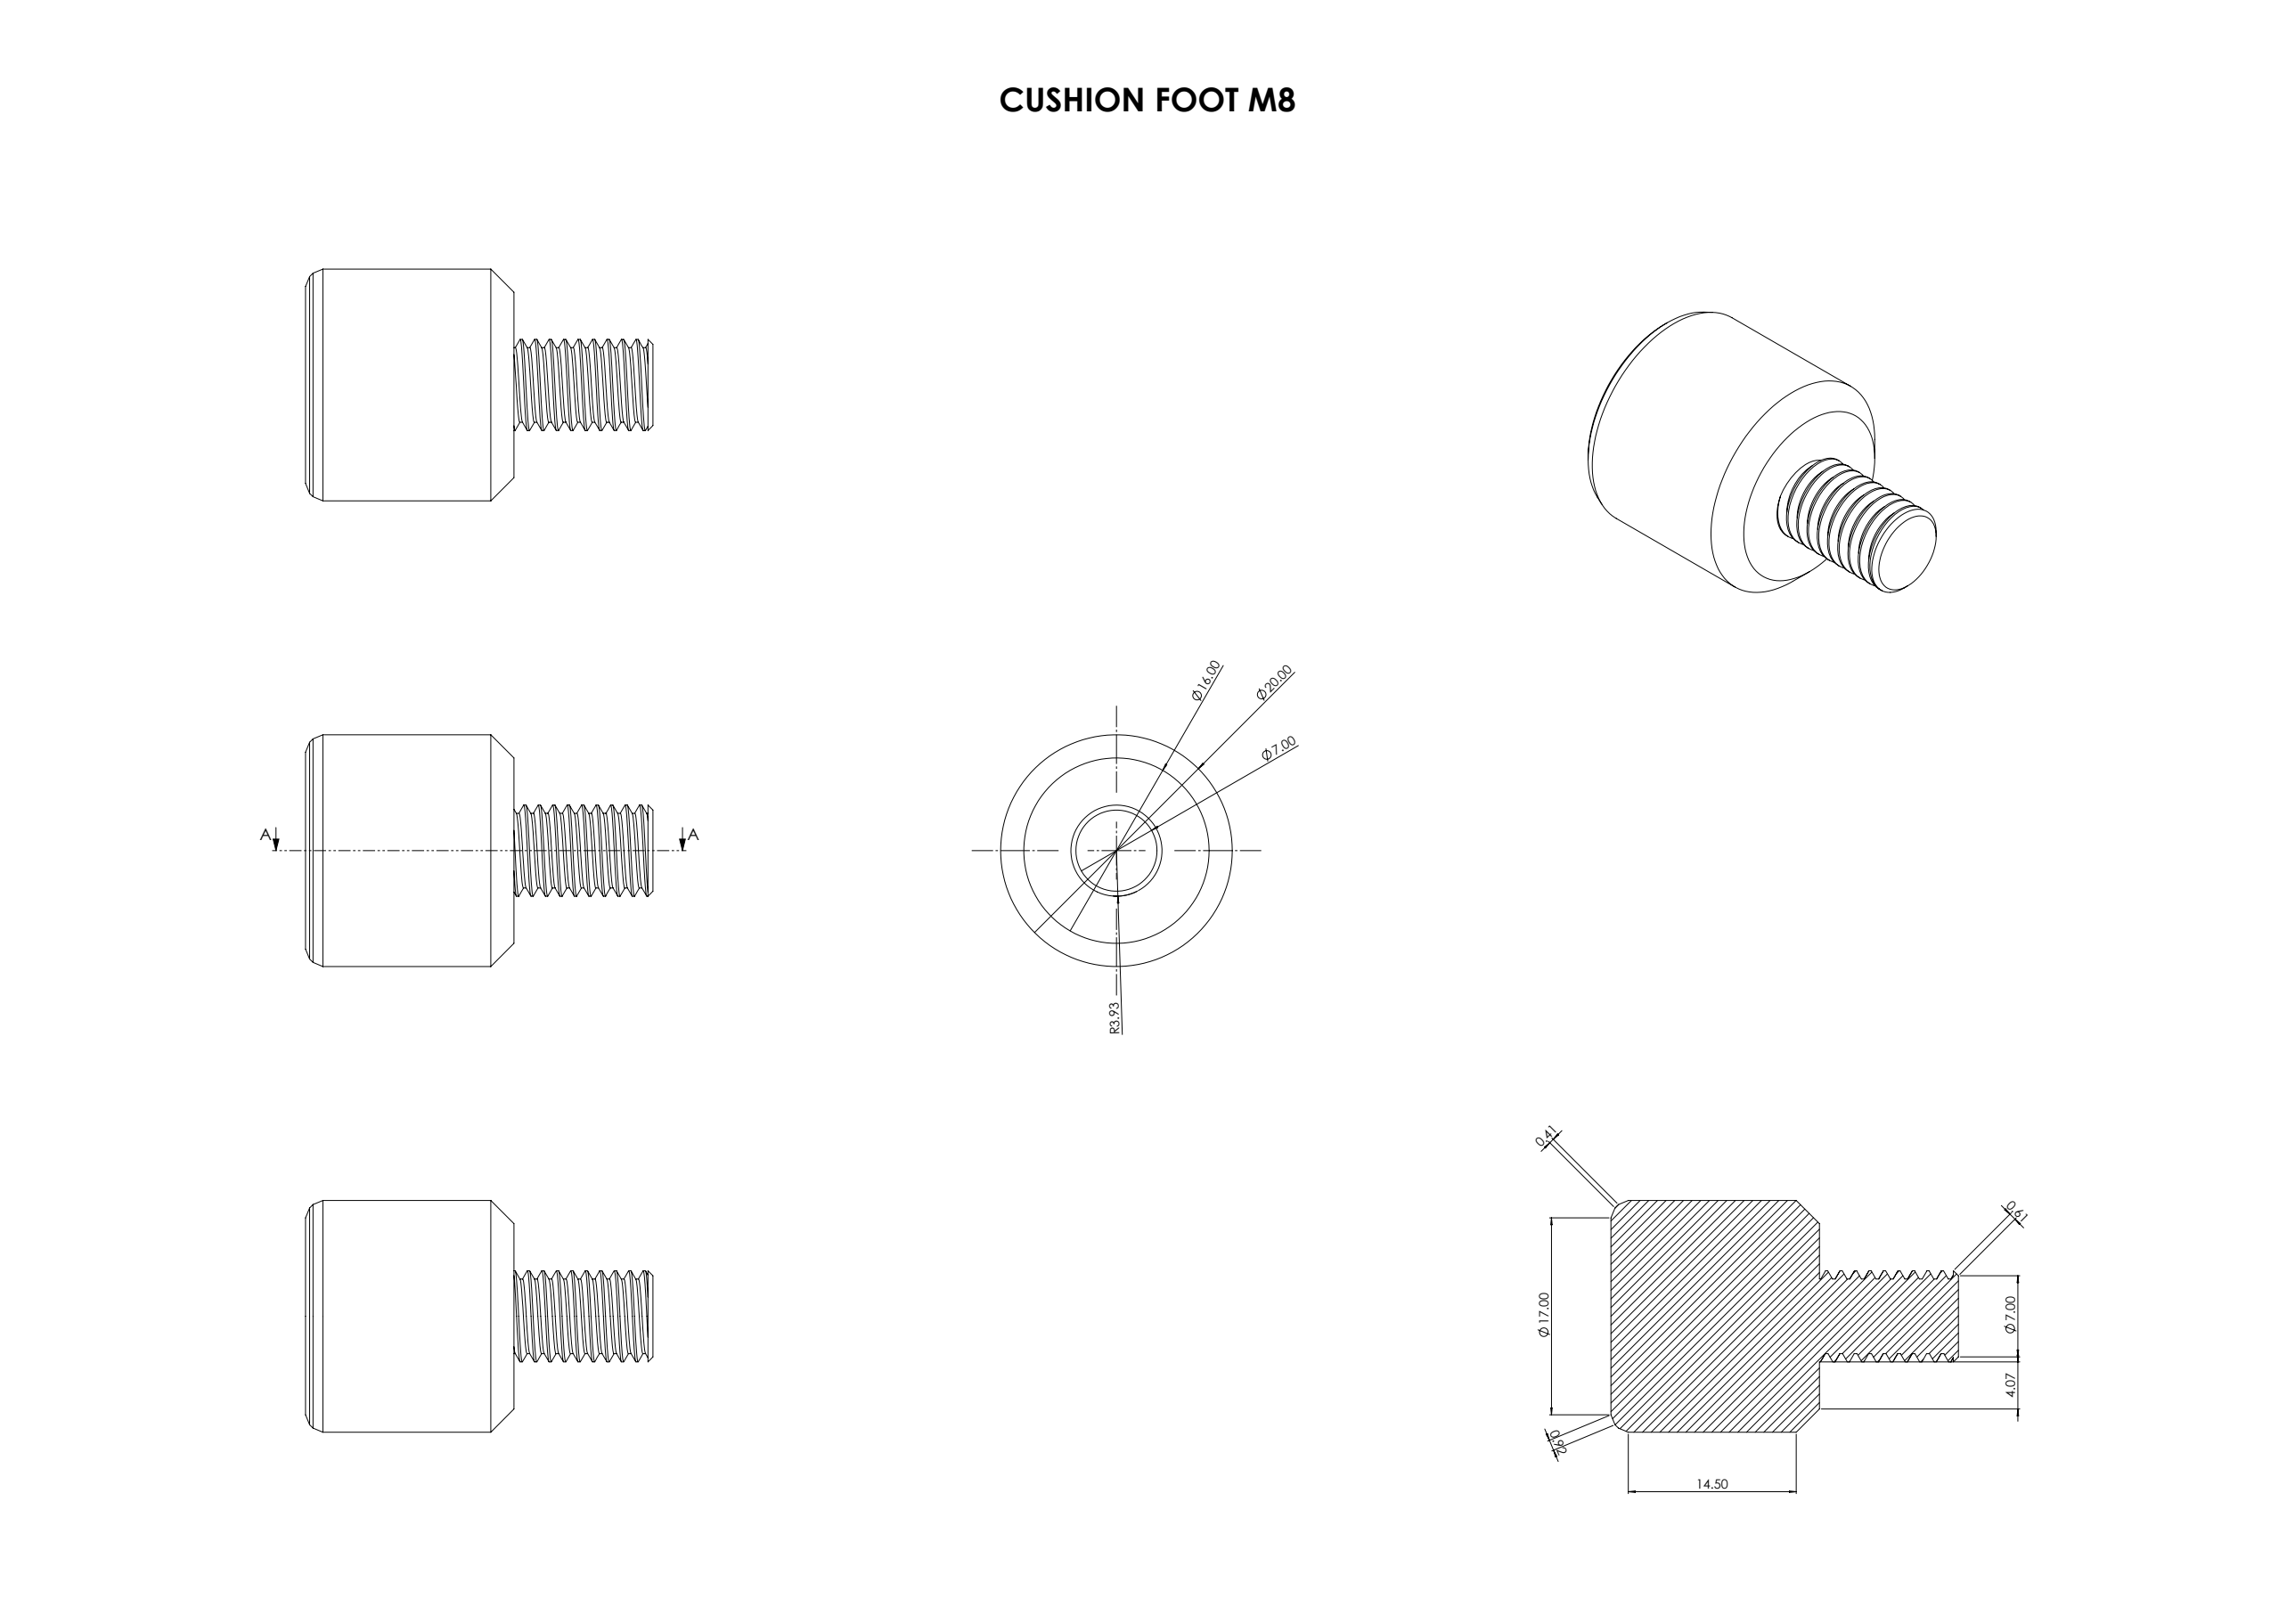
ISO-10303-21;
HEADER;
/* Generated by software containing ST-Developer
 * from STEP Tools, Inc. (www.steptools.com) 
 */

FILE_DESCRIPTION(
/* description */ (''),
/* implementation_level */ '2;1');

FILE_NAME(
/* name */ '15_Cushion_Foot_M8.step',
/* time_stamp */ '2026-10-26T06:13:19-07:00',
/* author */ (''),
/* organization */ (''),
/* preprocessor_version */ 'ST-DEVELOPER v20.2',
/* originating_system */ 'Autodesk Translation Framework v15.15.0.0',
/* authorisation */ '');

FILE_SCHEMA (('AUTOMOTIVE_DESIGN { 1 0 10303 214 3 1 1 }','TECHNICAL_DATA_PACKAGING'));
ENDSEC;

DATA;
#10=MECHANICAL_DESIGN_GEOMETRIC_PRESENTATION_REPRESENTATION('',(#313),#56639);
#273=SHAPE_REPRESENTATION_RELATIONSHIP('SRR','None',#56761,#293);
#293=ADVANCED_BREP_SHAPE_REPRESENTATION('',(#333),#56635);
#313=STYLED_ITEM('',(#56929),#333);
#333=MANIFOLD_SOLID_BREP('Body1',#16965);
#355=B_SPLINE_SURFACE_WITH_KNOTS('',3,3,((#37649,#37650,#37651,#37652,#37653,
#37654,#37655,#37656,#37657,#37658,#37659,#37660,#37661,#37662,#37663,#37664,
#37665,#37666,#37667,#37668,#37669,#37670,#37671,#37672,#37673,#37674,#37675,
#37676,#37677,#37678,#37679,#37680,#37681,#37682,#37683,#37684,#37685,#37686,
#37687,#37688,#37689,#37690,#37691,#37692,#37693,#37694,#37695,#37696,#37697,
#37698,#37699,#37700,#37701,#37702,#37703,#37704,#37705,#37706,#37707,#37708,
#37709,#37710,#37711,#37712),(#37713,#37714,#37715,#37716,#37717,#37718,
#37719,#37720,#37721,#37722,#37723,#37724,#37725,#37726,#37727,#37728,#37729,
#37730,#37731,#37732,#37733,#37734,#37735,#37736,#37737,#37738,#37739,#37740,
#37741,#37742,#37743,#37744,#37745,#37746,#37747,#37748,#37749,#37750,#37751,
#37752,#37753,#37754,#37755,#37756,#37757,#37758,#37759,#37760,#37761,#37762,
#37763,#37764,#37765,#37766,#37767,#37768,#37769,#37770,#37771,#37772,#37773,
#37774,#37775,#37776),(#37777,#37778,#37779,#37780,#37781,#37782,#37783,
#37784,#37785,#37786,#37787,#37788,#37789,#37790,#37791,#37792,#37793,#37794,
#37795,#37796,#37797,#37798,#37799,#37800,#37801,#37802,#37803,#37804,#37805,
#37806,#37807,#37808,#37809,#37810,#37811,#37812,#37813,#37814,#37815,#37816,
#37817,#37818,#37819,#37820,#37821,#37822,#37823,#37824,#37825,#37826,#37827,
#37828,#37829,#37830,#37831,#37832,#37833,#37834,#37835,#37836,#37837,#37838,
#37839,#37840),(#37841,#37842,#37843,#37844,#37845,#37846,#37847,#37848,
#37849,#37850,#37851,#37852,#37853,#37854,#37855,#37856,#37857,#37858,#37859,
#37860,#37861,#37862,#37863,#37864,#37865,#37866,#37867,#37868,#37869,#37870,
#37871,#37872,#37873,#37874,#37875,#37876,#37877,#37878,#37879,#37880,#37881,
#37882,#37883,#37884,#37885,#37886,#37887,#37888,#37889,#37890,#37891,#37892,
#37893,#37894,#37895,#37896,#37897,#37898,#37899,#37900,#37901,#37902,#37903,
#37904)),.UNSPECIFIED.,.F.,.F.,.F.,(4,4),(4,1,1,1,1,1,1,1,1,1,1,1,1,1,1,
1,1,1,1,1,1,1,1,1,1,1,1,1,1,1,1,1,1,1,1,1,1,1,1,1,1,1,1,1,1,1,1,1,1,1,1,
1,1,1,1,1,1,1,1,1,1,4),(0.,0.0820126057383863),(8.31473274985799,9.30167185077656,
10.2886109516951,11.2755500526137,12.2624891535323,13.2494282544508,14.2363673553694,
15.223306456288,16.2102455572066,17.1971846581251,18.1841237590437,19.1710628599623,
20.1580019608808,21.1449410617994,22.131880162718,23.1188192636365,24.1057583645551,
25.0926974654737,26.0796365663922,27.0665756673108,28.0535147682294,29.040453869148,
30.0273929700665,31.0143320709851,32.0012711719037,32.9882102728222,33.9751493737408,
34.9620884746594,35.9490275755779,36.9359666764965,37.9229057774151,38.9098448783337,
39.8967839792522,40.8837230801708,41.8706621810894,42.8576012820079,43.8445403829265,
44.8314794838451,45.8184185847636,46.8053576856822,47.7922967866008,48.7792358875193,
49.7661749884379,50.7531140893565,51.7400531902751,52.7269922911936,53.7139313921122,
54.7008704930308,55.6878095939493,56.6747486948679,57.6616877957865,58.6486268967051,
59.6355659976236,60.6225050985422,61.6094441994608,62.5963833003793,63.5833224012979,
64.5702615022165,65.557200603135,66.5441397040536,67.5310788049722,68.5180179058908),
 .UNSPECIFIED.);
#356=B_SPLINE_SURFACE_WITH_KNOTS('',3,3,((#38027,#38028,#38029,#38030,#38031,
#38032,#38033,#38034,#38035,#38036,#38037,#38038,#38039,#38040,#38041,#38042,
#38043,#38044,#38045,#38046,#38047,#38048,#38049,#38050,#38051,#38052,#38053,
#38054,#38055,#38056,#38057,#38058,#38059,#38060,#38061,#38062,#38063,#38064,
#38065,#38066,#38067,#38068,#38069,#38070,#38071,#38072,#38073,#38074,#38075,
#38076,#38077,#38078,#38079,#38080,#38081,#38082,#38083,#38084,#38085,#38086,
#38087,#38088,#38089,#38090),(#38091,#38092,#38093,#38094,#38095,#38096,
#38097,#38098,#38099,#38100,#38101,#38102,#38103,#38104,#38105,#38106,#38107,
#38108,#38109,#38110,#38111,#38112,#38113,#38114,#38115,#38116,#38117,#38118,
#38119,#38120,#38121,#38122,#38123,#38124,#38125,#38126,#38127,#38128,#38129,
#38130,#38131,#38132,#38133,#38134,#38135,#38136,#38137,#38138,#38139,#38140,
#38141,#38142,#38143,#38144,#38145,#38146,#38147,#38148,#38149,#38150,#38151,
#38152,#38153,#38154),(#38155,#38156,#38157,#38158,#38159,#38160,#38161,
#38162,#38163,#38164,#38165,#38166,#38167,#38168,#38169,#38170,#38171,#38172,
#38173,#38174,#38175,#38176,#38177,#38178,#38179,#38180,#38181,#38182,#38183,
#38184,#38185,#38186,#38187,#38188,#38189,#38190,#38191,#38192,#38193,#38194,
#38195,#38196,#38197,#38198,#38199,#38200,#38201,#38202,#38203,#38204,#38205,
#38206,#38207,#38208,#38209,#38210,#38211,#38212,#38213,#38214,#38215,#38216,
#38217,#38218),(#38219,#38220,#38221,#38222,#38223,#38224,#38225,#38226,
#38227,#38228,#38229,#38230,#38231,#38232,#38233,#38234,#38235,#38236,#38237,
#38238,#38239,#38240,#38241,#38242,#38243,#38244,#38245,#38246,#38247,#38248,
#38249,#38250,#38251,#38252,#38253,#38254,#38255,#38256,#38257,#38258,#38259,
#38260,#38261,#38262,#38263,#38264,#38265,#38266,#38267,#38268,#38269,#38270,
#38271,#38272,#38273,#38274,#38275,#38276,#38277,#38278,#38279,#38280,#38281,
#38282)),.UNSPECIFIED.,.F.,.F.,.F.,(4,4),(4,1,1,1,1,1,1,1,1,1,1,1,1,1,1,
1,1,1,1,1,1,1,1,1,1,1,1,1,1,1,1,1,1,1,1,1,1,1,1,1,1,1,1,1,1,1,1,1,1,1,1,
1,1,1,1,1,1,1,1,1,1,4),(0.,0.0820126057383863),(11.6152142277547,12.6021533286733,
13.5890924295918,14.5760315305104,15.562970631429,16.5499097323475,17.5368488332661,
18.5237879341847,19.5107270351033,20.4976661360218,21.4846052369404,22.471544337859,
23.4584834387775,24.4454225396961,25.4323616406147,26.4193007415332,27.4062398424518,
28.3931789433704,29.380118044289,30.3670571452075,31.3539962461261,32.3409353470447,
33.3278744479632,34.3148135488818,35.3017526498004,36.2886917507189,37.2756308516375,
38.2625699525561,39.2495090534747,40.2364481543932,41.2233872553118,42.2103263562304,
43.1972654571489,44.1842045580675,45.1711436589861,46.1580827599046,47.1450218608232,
48.1319609617418,49.1189000626604,50.1058391635789,51.0927782644975,52.0797173654161,
53.0666564663346,54.0535955672532,55.0405346681718,56.0274737690903,57.0144128700089,
58.0013519709275,58.9882910718461,59.9752301727646,60.9621692736832,61.9491083746018,
62.9360474755203,63.9229865764389,64.9099256773575,65.8968647782761,66.8838038791946,
67.8707429801132,68.8576820810318,69.8446211819503,70.8315602828689,71.8184993837875),
 .UNSPECIFIED.);
#559=FACE_BOUND('',#3561,.T.);
#643=CONICAL_SURFACE('',#18350,9.82322330470336,0.392699081698723);
#644=CONICAL_SURFACE('',#18355,9.5,0.785398163397448);
#645=CONICAL_SURFACE('',#18360,8.92677669529664,1.17809724509617);
#646=CONICAL_SURFACE('',#18369,9.,0.785398163397448);
#647=CONICAL_SURFACE('',#18372,3.75,0.785398163397451);
#1180=CIRCLE('',#18329,3.933);
#1181=CIRCLE('',#18339,3.933);
#1182=CIRCLE('',#18341,3.22275);
#1183=CIRCLE('',#18351,10.);
#1184=CIRCLE('',#18352,10.);
#1185=CIRCLE('',#18353,9.64644660940673);
#1186=CIRCLE('',#18354,9.64644660940673);
#1187=CIRCLE('',#18356,9.35355339059327);
#1188=CIRCLE('',#18357,9.35355339059327);
#1189=CIRCLE('',#18359,10.);
#1190=CIRCLE('',#18361,8.5);
#1191=CIRCLE('',#18364,3.933);
#1192=CIRCLE('',#18366,3.22275);
#1193=CIRCLE('',#18368,3.933);
#1194=CIRCLE('',#18370,8.);
#1195=CIRCLE('',#18373,3.5);
#1470=CYLINDRICAL_SURFACE('',#18328,3.933);
#1471=CYLINDRICAL_SURFACE('',#18330,3.933);
#1472=CYLINDRICAL_SURFACE('',#18331,3.933);
#1473=CYLINDRICAL_SURFACE('',#18332,3.933);
#1474=CYLINDRICAL_SURFACE('',#18333,3.933);
#1475=CYLINDRICAL_SURFACE('',#18334,3.933);
#1476=CYLINDRICAL_SURFACE('',#18335,3.933);
#1477=CYLINDRICAL_SURFACE('',#18336,3.933);
#1478=CYLINDRICAL_SURFACE('',#18337,3.933);
#1479=CYLINDRICAL_SURFACE('',#18338,3.933);
#1480=CYLINDRICAL_SURFACE('',#18340,3.22275);
#1481=CYLINDRICAL_SURFACE('',#18342,3.22275);
#1482=CYLINDRICAL_SURFACE('',#18343,3.22275);
#1483=CYLINDRICAL_SURFACE('',#18344,3.22275);
#1484=CYLINDRICAL_SURFACE('',#18345,3.22275);
#1485=CYLINDRICAL_SURFACE('',#18346,3.22275);
#1486=CYLINDRICAL_SURFACE('',#18347,3.22275);
#1487=CYLINDRICAL_SURFACE('',#18348,3.22275);
#1488=CYLINDRICAL_SURFACE('',#18349,3.22275);
#1489=CYLINDRICAL_SURFACE('',#18358,10.);
#1490=CYLINDRICAL_SURFACE('',#18365,3.22275);
#1491=CYLINDRICAL_SURFACE('',#18367,3.933);
#2412=FACE_OUTER_BOUND('',#3530,.T.);
#2413=FACE_OUTER_BOUND('',#3531,.T.);
#2414=FACE_OUTER_BOUND('',#3532,.T.);
#2415=FACE_OUTER_BOUND('',#3533,.T.);
#2416=FACE_OUTER_BOUND('',#3534,.T.);
#2417=FACE_OUTER_BOUND('',#3535,.T.);
#2418=FACE_OUTER_BOUND('',#3536,.T.);
#2419=FACE_OUTER_BOUND('',#3537,.T.);
#2420=FACE_OUTER_BOUND('',#3538,.T.);
#2421=FACE_OUTER_BOUND('',#3539,.T.);
#2422=FACE_OUTER_BOUND('',#3540,.T.);
#2423=FACE_OUTER_BOUND('',#3541,.T.);
#2424=FACE_OUTER_BOUND('',#3542,.T.);
#2425=FACE_OUTER_BOUND('',#3543,.T.);
#2426=FACE_OUTER_BOUND('',#3544,.T.);
#2427=FACE_OUTER_BOUND('',#3545,.T.);
#2428=FACE_OUTER_BOUND('',#3546,.T.);
#2429=FACE_OUTER_BOUND('',#3547,.T.);
#2430=FACE_OUTER_BOUND('',#3548,.T.);
#2431=FACE_OUTER_BOUND('',#3549,.T.);
#2432=FACE_OUTER_BOUND('',#3550,.T.);
#2433=FACE_OUTER_BOUND('',#3551,.T.);
#2434=FACE_OUTER_BOUND('',#3552,.T.);
#2435=FACE_OUTER_BOUND('',#3553,.T.);
#2436=FACE_OUTER_BOUND('',#3554,.T.);
#2437=FACE_OUTER_BOUND('',#3555,.T.);
#2438=FACE_OUTER_BOUND('',#3556,.T.);
#2439=FACE_OUTER_BOUND('',#3557,.T.);
#2440=FACE_OUTER_BOUND('',#3558,.T.);
#2441=FACE_OUTER_BOUND('',#3559,.T.);
#2442=FACE_OUTER_BOUND('',#3560,.T.);
#2443=FACE_OUTER_BOUND('',#3562,.T.);
#2444=FACE_OUTER_BOUND('',#3563,.T.);
#3530=EDGE_LOOP('',(#13640,#13641,#13642,#13643));
#3531=EDGE_LOOP('',(#13644,#13645,#13646,#13647));
#3532=EDGE_LOOP('',(#13648,#13649,#13650,#13651));
#3533=EDGE_LOOP('',(#13652,#13653,#13654,#13655));
#3534=EDGE_LOOP('',(#13656,#13657,#13658,#13659));
#3535=EDGE_LOOP('',(#13660,#13661,#13662,#13663));
#3536=EDGE_LOOP('',(#13664,#13665,#13666,#13667));
#3537=EDGE_LOOP('',(#13668,#13669,#13670,#13671));
#3538=EDGE_LOOP('',(#13672,#13673,#13674,#13675));
#3539=EDGE_LOOP('',(#13676,#13677,#13678,#13679,#13680));
#3540=EDGE_LOOP('',(#13681,#13682,#13683,#13684));
#3541=EDGE_LOOP('',(#13685,#13686,#13687,#13688));
#3542=EDGE_LOOP('',(#13689,#13690,#13691,#13692));
#3543=EDGE_LOOP('',(#13693,#13694,#13695,#13696));
#3544=EDGE_LOOP('',(#13697,#13698,#13699,#13700));
#3545=EDGE_LOOP('',(#13701,#13702,#13703,#13704));
#3546=EDGE_LOOP('',(#13705,#13706,#13707,#13708));
#3547=EDGE_LOOP('',(#13709,#13710,#13711,#13712));
#3548=EDGE_LOOP('',(#13713,#13714,#13715,#13716));
#3549=EDGE_LOOP('',(#13717,#13718,#13719,#13720,#13721,#13722));
#3550=EDGE_LOOP('',(#13723,#13724,#13725,#13726,#13727,#13728));
#3551=EDGE_LOOP('',(#13729,#13730,#13731,#13732,#13733));
#3552=EDGE_LOOP('',(#13734,#13735,#13736,#13737,#13738));
#3553=EDGE_LOOP('',(#13739));
#3554=EDGE_LOOP('',(#13740,#13741,#13742,#13743));
#3555=EDGE_LOOP('',(#13744,#13745,#13746,#13747,#13748,#13749,#13750,#13751,
#13752,#13753,#13754,#13755,#13756,#13757,#13758,#13759,#13760,#13761,#13762,
#13763,#13764,#13765,#13766));
#3556=EDGE_LOOP('',(#13767,#13768,#13769,#13770));
#3557=EDGE_LOOP('',(#13771,#13772,#13773,#13774,#13775,#13776,#13777,#13778,
#13779,#13780,#13781,#13782,#13783,#13784,#13785,#13786,#13787,#13788,#13789,
#13790,#13791,#13792));
#3558=EDGE_LOOP('',(#13793,#13794,#13795));
#3559=EDGE_LOOP('',(#13796,#13797,#13798,#13799));
#3560=EDGE_LOOP('',(#13800));
#3561=EDGE_LOOP('',(#13801,#13802,#13803,#13804));
#3562=EDGE_LOOP('',(#13805,#13806,#13807,#13808,#13809,#13810));
#3563=EDGE_LOOP('',(#13811));
#4515=LINE('',#36739,#5469);
#4516=LINE('',#36763,#5470);
#4517=LINE('',#36811,#5471);
#4518=LINE('',#36859,#5472);
#4519=LINE('',#36913,#5473);
#4520=LINE('',#36961,#5474);
#4521=LINE('',#37009,#5475);
#4522=LINE('',#37063,#5476);
#4523=LINE('',#37111,#5477);
#4524=LINE('',#37165,#5478);
#4525=LINE('',#37212,#5479);
#4526=LINE('',#37232,#5480);
#4527=LINE('',#37257,#5481);
#4528=LINE('',#37282,#5482);
#4529=LINE('',#37307,#5483);
#4530=LINE('',#37332,#5484);
#4531=LINE('',#37356,#5485);
#4532=LINE('',#37381,#5486);
#4533=LINE('',#37406,#5487);
#4534=LINE('',#37433,#5488);
#4535=LINE('',#37439,#5489);
#4536=LINE('',#37446,#5490);
#4537=LINE('',#37449,#5491);
#4538=LINE('',#38385,#5492);
#4539=LINE('',#38390,#5493);
#5469=VECTOR('',#21681,4.);
#5470=VECTOR('',#21686,4.);
#5471=VECTOR('',#21689,4.);
#5472=VECTOR('',#21692,4.);
#5473=VECTOR('',#21695,4.);
#5474=VECTOR('',#21698,4.);
#5475=VECTOR('',#21701,4.);
#5476=VECTOR('',#21704,4.);
#5477=VECTOR('',#21707,4.);
#5478=VECTOR('',#21710,4.);
#5479=VECTOR('',#21715,3.22275);
#5480=VECTOR('',#21720,3.22275);
#5481=VECTOR('',#21723,3.22275);
#5482=VECTOR('',#21726,3.22275);
#5483=VECTOR('',#21729,3.22275);
#5484=VECTOR('',#21732,3.22275);
#5485=VECTOR('',#21735,3.22275);
#5486=VECTOR('',#21738,3.22275);
#5487=VECTOR('',#21741,3.22275);
#5488=VECTOR('',#21748,9.82322330470336);
#5489=VECTOR('',#21755,9.5);
#5490=VECTOR('',#21764,10.);
#5491=VECTOR('',#21767,8.92677669529664);
#5492=VECTOR('',#21788,9.);
#5493=VECTOR('',#21795,3.75);
#6085=B_SPLINE_CURVE_WITH_KNOTS('',3,(#36741,#36742,#36743,#36744,#36745,
#36746,#36747,#36748,#36749,#36750),.UNSPECIFIED.,.F.,.F.,(4,3,3,4),(-4.09274904019423,
-3.94775640367428,-2.96081730275571,-2.06120159751578),.UNSPECIFIED.);
#6086=B_SPLINE_CURVE_WITH_KNOTS('',3,(#36753,#36754,#36755,#36756,#36757,
#36758,#36759),.UNSPECIFIED.,.F.,.F.,(4,3,4),(0.,0.986939100918566,1.11004521091131),
 .UNSPECIFIED.);
#6087=B_SPLINE_CURVE_WITH_KNOTS('',3,(#36764,#36765,#36766,#36767,#36768,
#36769,#36770,#36771,#36772,#36773,#36774,#36775,#36776,#36777,#36778,#36779,
#36780,#36781,#36782,#36783,#36784,#36785),.UNSPECIFIED.,.F.,.F.,(4,3,3,
3,3,3,3,4),(-10.3759343473738,-9.8693910091857,-8.88245190826713,-7.89551280734856,
-6.90857370642999,-5.92163460551142,-4.93469550459285,-4.09274904019423),
 .UNSPECIFIED.);
#6088=B_SPLINE_CURVE_WITH_KNOTS('',3,(#36786,#36787,#36788,#36789,#36790,
#36791,#36792,#36793,#36794,#36795,#36796,#36797,#36798,#36799,#36800,#36801,
#36802,#36803,#36804,#36805,#36806,#36807),.UNSPECIFIED.,.F.,.F.,(4,3,3,
3,3,3,3,4),(1.11004521091131,1.97387820183714,2.96081730275571,3.94775640367428,
4.93469550459285,5.92163460551142,6.90857370642999,7.39323051809089),
 .UNSPECIFIED.);
#6089=B_SPLINE_CURVE_WITH_KNOTS('',3,(#36812,#36813,#36814,#36815,#36816,
#36817,#36818,#36819,#36820,#36821,#36822,#36823,#36824,#36825,#36826,#36827,
#36828,#36829,#36830,#36831,#36832,#36833),.UNSPECIFIED.,.F.,.F.,(4,3,3,
3,3,3,3,4),(-16.6591196545534,-15.7910256146971,-14.8040865137786,-13.81714741286,
-12.8302083119414,-11.8432692110228,-10.8563301101043,-10.3759343473738),
 .UNSPECIFIED.);
#6090=B_SPLINE_CURVE_WITH_KNOTS('',3,(#36834,#36835,#36836,#36837,#36838,
#36839,#36840,#36841,#36842,#36843,#36844,#36845,#36846,#36847,#36848,#36849,
#36850,#36851,#36852,#36853,#36854,#36855),.UNSPECIFIED.,.F.,.F.,(4,3,3,
3,3,3,3,4),(7.39323051809089,7.89551280734856,8.88245190826713,9.8693910091857,
10.8563301101043,11.8432692110228,12.8302083119414,13.6764158252705),
 .UNSPECIFIED.);
#6091=B_SPLINE_CURVE_WITH_KNOTS('',3,(#36860,#36861,#36862,#36863,#36864,
#36865,#36866,#36867,#36868,#36869,#36870,#36871,#36872,#36873,#36874,#36875,
#36876,#36877,#36878,#36879,#36880,#36881,#36882,#36883,#36884),
 .UNSPECIFIED.,.F.,.F.,(4,3,3,3,3,3,3,3,4),(-22.942304961733,-22.6995993211271,
-21.7126602202085,-20.72572111929,-19.7387820183714,-18.7518429174528,-17.7649038165343,
-16.7779647156157,-16.6591196545534),.UNSPECIFIED.);
#6092=B_SPLINE_CURVE_WITH_KNOTS('',3,(#36885,#36886,#36887,#36888,#36889,
#36890,#36891,#36892,#36893,#36894,#36895,#36896,#36897,#36898,#36899,#36900,
#36901,#36902,#36903,#36904,#36905,#36906,#36907,#36908,#36909),
 .UNSPECIFIED.,.F.,.F.,(4,3,3,3,3,3,3,3,4),(13.6764158252705,13.81714741286,
14.8040865137786,15.7910256146971,16.7779647156157,17.7649038165343,18.7518429174528,
19.7387820183714,19.9596011324501),.UNSPECIFIED.);
#6093=B_SPLINE_CURVE_WITH_KNOTS('',3,(#36914,#36915,#36916,#36917,#36918,
#36919,#36920,#36921,#36922,#36923,#36924,#36925,#36926,#36927,#36928,#36929,
#36930,#36931,#36932,#36933,#36934,#36935),.UNSPECIFIED.,.F.,.F.,(4,3,3,
3,3,3,3,4),(-29.2254902689126,-28.6212339266385,-27.63429482572,-26.6473557248014,
-25.6604166238828,-24.6734775229643,-23.6865384220457,-22.942304961733),
 .UNSPECIFIED.);
#6094=B_SPLINE_CURVE_WITH_KNOTS('',3,(#36936,#36937,#36938,#36939,#36940,
#36941,#36942,#36943,#36944,#36945,#36946,#36947,#36948,#36949,#36950,#36951,
#36952,#36953,#36954,#36955,#36956,#36957),.UNSPECIFIED.,.F.,.F.,(4,3,3,
3,3,3,3,4),(19.9596011324501,20.72572111929,21.7126602202085,22.6995993211271,
23.6865384220457,24.6734775229642,25.6604166238828,26.2427864396297),
 .UNSPECIFIED.);
#6095=B_SPLINE_CURVE_WITH_KNOTS('',3,(#36962,#36963,#36964,#36965,#36966,
#36967,#36968,#36969,#36970,#36971,#36972,#36973,#36974,#36975,#36976,#36977,
#36978,#36979,#36980,#36981,#36982,#36983),.UNSPECIFIED.,.F.,.F.,(4,3,3,
3,3,3,3,4),(-35.5086755760922,-34.54286853215,-33.5559294312314,-32.5689903303128,
-31.5820512293942,-30.5951121284757,-29.6081730275571,-29.2254902689126),
 .UNSPECIFIED.);
#6096=B_SPLINE_CURVE_WITH_KNOTS('',3,(#36984,#36985,#36986,#36987,#36988,
#36989,#36990,#36991,#36992,#36993,#36994,#36995,#36996,#36997,#36998,#36999,
#37000,#37001,#37002,#37003,#37004,#37005),.UNSPECIFIED.,.F.,.F.,(4,3,3,
3,3,3,3,4),(26.2427864396297,26.6473557248014,27.63429482572,28.6212339266385,
29.6081730275571,30.5951121284757,31.5820512293942,32.5259717468092),
 .UNSPECIFIED.);
#6097=B_SPLINE_CURVE_WITH_KNOTS('',3,(#37010,#37011,#37012,#37013,#37014,
#37015,#37016,#37017,#37018,#37019,#37020,#37021,#37022,#37023,#37024,#37025,
#37026,#37027,#37028,#37029,#37030,#37031,#37032,#37033,#37034),
 .UNSPECIFIED.,.F.,.F.,(4,3,3,3,3,3,3,3,4),(-41.7918608832717,-41.4514422385799,
-40.4645031376614,-39.4775640367428,-38.4906249358242,-37.5036858349057,
-36.5167467339871,-35.5298076330685,-35.5086755760922),.UNSPECIFIED.);
#6098=B_SPLINE_CURVE_WITH_KNOTS('',3,(#37035,#37036,#37037,#37038,#37039,
#37040,#37041,#37042,#37043,#37044,#37045,#37046,#37047,#37048,#37049,#37050,
#37051,#37052,#37053,#37054,#37055,#37056,#37057,#37058,#37059),
 .UNSPECIFIED.,.F.,.F.,(4,3,3,3,3,3,3,3,4),(32.5259717468092,32.5689903303128,
33.5559294312314,34.54286853215,35.5298076330685,36.5167467339871,37.5036858349057,
38.4906249358242,38.8091570539888),.UNSPECIFIED.);
#6099=B_SPLINE_CURVE_WITH_KNOTS('',3,(#37064,#37065,#37066,#37067,#37068,
#37069,#37070,#37071,#37072,#37073,#37074,#37075,#37076,#37077,#37078,#37079,
#37080,#37081,#37082,#37083,#37084,#37085),.UNSPECIFIED.,.F.,.F.,(4,3,3,
3,3,3,3,4),(-48.0750461904514,-47.3730768440914,-46.3861377431728,-45.3991986422542,
-44.4122595413357,-43.4253204404171,-42.4383813394985,-41.7918608832717),
 .UNSPECIFIED.);
#6100=B_SPLINE_CURVE_WITH_KNOTS('',3,(#37086,#37087,#37088,#37089,#37090,
#37091,#37092,#37093,#37094,#37095,#37096,#37097,#37098,#37099,#37100,#37101,
#37102,#37103,#37104,#37105,#37106,#37107),.UNSPECIFIED.,.F.,.F.,(4,3,3,
3,3,3,3,4),(38.8091570539888,39.4775640367428,40.4645031376614,41.4514422385799,
42.4383813394985,43.4253204404171,44.4122595413357,45.0923423611684),
 .UNSPECIFIED.);
#6101=B_SPLINE_CURVE_WITH_KNOTS('',3,(#37112,#37113,#37114,#37115,#37116,
#37117,#37118,#37119,#37120,#37121,#37122,#37123,#37124,#37125,#37126,#37127,
#37128,#37129,#37130,#37131,#37132,#37133,#37134,#37135,#37136),
 .UNSPECIFIED.,.F.,.F.,(4,3,3,3,3,3,3,3,4),(-54.3582314976309,-54.2816505505214,
-53.2947114496028,-52.3077723486842,-51.3208332477656,-50.3338941468471,
-49.3469550459285,-48.3600159450099,-48.0750461904514),.UNSPECIFIED.);
#6102=B_SPLINE_CURVE_WITH_KNOTS('',3,(#37137,#37138,#37139,#37140,#37141,
#37142,#37143,#37144,#37145,#37146,#37147,#37148,#37149,#37150,#37151,#37152,
#37153,#37154,#37155,#37156,#37157,#37158,#37159,#37160,#37161),
 .UNSPECIFIED.,.F.,.F.,(4,3,3,3,3,3,3,3,4),(45.0923423611684,45.3991986422542,
46.3861377431728,47.3730768440914,48.3600159450099,49.3469550459285,50.3338941468471,
51.3208332477656,51.375527668348),.UNSPECIFIED.);
#6103=B_SPLINE_CURVE_WITH_KNOTS('',3,(#37168,#37169,#37170,#37171,#37172,
#37173,#37174,#37175,#37176,#37177,#37178,#37179,#37180,#37181,#37182,#37183,
#37184,#37185,#37186),.UNSPECIFIED.,.F.,.F.,(4,3,3,3,3,3,4),(-60.2032851560328,
-59.2163460551142,-58.2294069541956,-57.2424678532771,-56.2555287523585,
-55.2685896514399,-54.3582314976309),.UNSPECIFIED.);
#6104=B_SPLINE_CURVE_WITH_KNOTS('',3,(#37187,#37188,#37189,#37190,#37191,
#37192,#37193,#37194,#37195,#37196,#37197,#37198,#37199,#37200,#37201,#37202,
#37203,#37204,#37205,#37206,#37207,#37208),.UNSPECIFIED.,.F.,.F.,(4,3,3,
3,3,3,3,4),(51.375527668348,52.3077723486842,53.2947114496028,54.2816505505213,
55.2685896514399,56.2555287523585,57.242467853277,57.6587129755276),
 .UNSPECIFIED.);
#6105=B_SPLINE_CURVE_WITH_KNOTS('',3,(#37214,#37215,#37216,#37217,#37218,
#37219,#37220),.UNSPECIFIED.,.F.,.F.,(4,1,1,1,4),(65.9734457253856,66.8838038791946,
67.8707429801132,68.8576820810318,69.7572977862717),.UNSPECIFIED.);
#6106=B_SPLINE_CURVE_WITH_KNOTS('',3,(#37223,#37224,#37225,#37226,#37227,
#37228),.UNSPECIFIED.,.F.,.F.,(4,1,1,4),(65.9734457253856,66.5441397040536,
67.5310788049722,68.5180179058908),.UNSPECIFIED.);
#6107=B_SPLINE_CURVE_WITH_KNOTS('',3,(#37233,#37234,#37235,#37236,#37237,
#37238,#37239,#37240,#37241,#37242,#37243),.UNSPECIFIED.,.F.,.F.,(4,1,1,
1,1,1,1,1,4),(59.6902604182061,59.9752301727646,60.9621692736832,61.9491083746018,
62.9360474755203,63.9229865764389,64.9099256773575,65.8968647782761,65.9734457253856),
 .UNSPECIFIED.);
#6108=B_SPLINE_CURVE_WITH_KNOTS('',3,(#37244,#37245,#37246,#37247,#37248,
#37249,#37250,#37251,#37252,#37253),.UNSPECIFIED.,.F.,.F.,(4,1,1,1,1,1,
1,4),(59.6902604182061,60.6225050985422,61.6094441994608,62.5963833003793,
63.5833224012979,64.5702615022165,65.557200603135,65.9734457253856),
 .UNSPECIFIED.);
#6109=B_SPLINE_CURVE_WITH_KNOTS('',3,(#37258,#37259,#37260,#37261,#37262,
#37263,#37264,#37265,#37266,#37267),.UNSPECIFIED.,.F.,.F.,(4,1,1,1,1,1,
1,4),(53.4070751110265,54.0535955672532,55.0405346681718,56.0274737690903,
57.0144128700089,58.0013519709275,58.9882910718461,59.6902604182061),
 .UNSPECIFIED.);
#6110=B_SPLINE_CURVE_WITH_KNOTS('',3,(#37268,#37269,#37270,#37271,#37272,
#37273,#37274,#37275,#37276,#37277,#37278),.UNSPECIFIED.,.F.,.F.,(4,1,1,
1,1,1,1,1,4),(53.4070751110265,53.7139313921122,54.7008704930308,55.6878095939493,
56.6747486948679,57.6616877957865,58.6486268967051,59.6355659976236,59.6902604182061),
 .UNSPECIFIED.);
#6111=B_SPLINE_CURVE_WITH_KNOTS('',3,(#37283,#37284,#37285,#37286,#37287,
#37288,#37289,#37290,#37291,#37292,#37293),.UNSPECIFIED.,.F.,.F.,(4,1,1,
1,1,1,1,1,4),(47.1238898038469,47.1450218608232,48.1319609617418,49.1189000626604,
50.1058391635789,51.0927782644975,52.0797173654161,53.0666564663346,53.4070751110265),
 .UNSPECIFIED.);
#6112=B_SPLINE_CURVE_WITH_KNOTS('',3,(#37294,#37295,#37296,#37297,#37298,
#37299,#37300,#37301,#37302,#37303),.UNSPECIFIED.,.F.,.F.,(4,1,1,1,1,1,
1,4),(47.1238898038469,47.7922967866008,48.7792358875193,49.7661749884379,
50.7531140893565,51.7400531902751,52.7269922911936,53.4070751110265),
 .UNSPECIFIED.);
#6113=B_SPLINE_CURVE_WITH_KNOTS('',3,(#37308,#37309,#37310,#37311,#37312,
#37313,#37314,#37315,#37316,#37317),.UNSPECIFIED.,.F.,.F.,(4,1,1,1,1,1,
1,4),(40.8407044966673,41.2233872553118,42.2103263562304,43.1972654571489,
44.1842045580675,45.1711436589861,46.1580827599046,47.1238898038469),
 .UNSPECIFIED.);
#6114=B_SPLINE_CURVE_WITH_KNOTS('',3,(#37318,#37319,#37320,#37321,#37322,
#37323,#37324,#37325,#37326,#37327,#37328),.UNSPECIFIED.,.F.,.F.,(4,1,1,
1,1,1,1,1,4),(40.8407044966673,40.8837230801708,41.8706621810894,42.8576012820079,
43.8445403829265,44.8314794838451,45.8184185847636,46.8053576856822,47.1238898038469),
 .UNSPECIFIED.);
#6115=B_SPLINE_CURVE_WITH_KNOTS('',3,(#37333,#37334,#37335,#37336,#37337,
#37338,#37339,#37340,#37341,#37342),.UNSPECIFIED.,.F.,.F.,(4,1,1,1,1,1,
1,4),(34.5575191894877,35.3017526498004,36.2886917507189,37.2756308516375,
38.2625699525561,39.2495090534747,40.2364481543932,40.8407044966673),
 .UNSPECIFIED.);
#6116=B_SPLINE_CURVE_WITH_KNOTS('',3,(#37343,#37344,#37345,#37346,#37347,
#37348,#37349,#37350,#37351,#37352),.UNSPECIFIED.,.F.,.F.,(4,1,1,1,1,1,
1,4),(34.5575191894877,34.9620884746594,35.9490275755779,36.9359666764965,
37.9229057774151,38.9098448783337,39.8967839792522,40.8407044966673),
 .UNSPECIFIED.);
#6117=B_SPLINE_CURVE_WITH_KNOTS('',3,(#37357,#37358,#37359,#37360,#37361,
#37362,#37363,#37364,#37365,#37366,#37367),.UNSPECIFIED.,.F.,.F.,(4,1,1,
1,1,1,1,1,4),(28.2743338823081,28.3931789433704,29.380118044289,30.3670571452075,
31.3539962461261,32.3409353470447,33.3278744479632,34.3148135488818,34.5575191894877),
 .UNSPECIFIED.);
#6118=B_SPLINE_CURVE_WITH_KNOTS('',3,(#37368,#37369,#37370,#37371,#37372,
#37373,#37374,#37375,#37376,#37377),.UNSPECIFIED.,.F.,.F.,(4,1,1,1,1,1,
1,4),(28.2743338823081,29.040453869148,30.0273929700665,31.0143320709851,
32.0012711719037,32.9882102728222,33.9751493737408,34.5575191894877),
 .UNSPECIFIED.);
#6119=B_SPLINE_CURVE_WITH_KNOTS('',3,(#37382,#37383,#37384,#37385,#37386,
#37387,#37388,#37389,#37390,#37391),.UNSPECIFIED.,.F.,.F.,(4,1,1,1,1,1,
1,4),(21.9911485751285,22.471544337859,23.4584834387775,24.4454225396961,
25.4323616406147,26.4193007415332,27.4062398424518,28.2743338823081),
 .UNSPECIFIED.);
#6120=B_SPLINE_CURVE_WITH_KNOTS('',3,(#37392,#37393,#37394,#37395,#37396,
#37397,#37398,#37399,#37400,#37401,#37402),.UNSPECIFIED.,.F.,.F.,(4,1,1,
1,1,1,1,1,4),(21.9911485751285,22.131880162718,23.1188192636365,24.1057583645551,
25.0926974654737,26.0796365663922,27.0665756673108,28.0535147682294,28.2743338823081),
 .UNSPECIFIED.);
#6121=B_SPLINE_CURVE_WITH_KNOTS('',3,(#37407,#37408,#37409,#37410,#37411,
#37412,#37413,#37414,#37415,#37416),.UNSPECIFIED.,.F.,.F.,(4,1,1,1,1,1,
1,4),(15.7079632679489,16.5499097323475,17.5368488332661,18.5237879341847,
19.5107270351033,20.4976661360218,21.4846052369404,21.9911485751285),
 .UNSPECIFIED.);
#6122=B_SPLINE_CURVE_WITH_KNOTS('',3,(#37417,#37418,#37419,#37420,#37421,
#37422,#37423,#37424,#37425,#37426),.UNSPECIFIED.,.F.,.F.,(4,1,1,1,1,1,
1,4),(15.7079632679489,16.2102455572066,17.1971846581251,18.1841237590437,
19.1710628599623,20.1580019608808,21.1449410617994,21.9911485751285),
 .UNSPECIFIED.);
#6123=B_SPLINE_CURVE_WITH_KNOTS('',3,(#37453,#37454,#37455,#37456,#37457,
#37458,#37459,#37460,#37461,#37462,#37463,#37464,#37465,#37466,#37467,#37468,
#37469,#37470,#37471,#37472,#37473,#37474,#37475,#37476,#37477,#37478,#37479,
#37480,#37481,#37482,#37483,#37484,#37485,#37486,#37487,#37488,#37489,#37490,
#37491,#37492,#37493,#37494,#37495,#37496,#37497,#37498,#37499,#37500,#37501,
#37502,#37503,#37504,#37505,#37506,#37507,#37508,#37509,#37510,#37511,#37512,
#37513,#37514,#37515,#37516,#37517,#37518,#37519,#37520,#37521,#37522,#37523,
#37524,#37525,#37526,#37527,#37528,#37529,#37530,#37531,#37532,#37533,#37534,
#37535,#37536,#37537,#37538,#37539,#37540,#37541,#37542,#37543,#37544,#37545,
#37546,#37547,#37548,#37549),.UNSPECIFIED.,.F.,.F.,(4,3,3,3,3,3,3,3,3,3,
3,3,3,3,3,3,3,3,3,3,3,3,3,3,3,3,3,3,3,3,3,3,4),(-0.744397949170625,-0.71583061742043,
-0.684607549726404,-0.665225811669408,-0.65913755838546,-0.653541781901175,
-0.621561581432833,-0.590678851355536,-0.576678185830625,-0.57109179287764,
-0.537836542473585,-0.504009698787253,-0.47015729823496,-0.446242908879834,
-0.439103797305219,-0.43297135889342,-0.398062560014724,-0.374499740814454,
-0.340715815821642,-0.306315596621499,-0.298239329175978,-0.292491744365664,
-0.258101152324883,-0.222604526272566,-0.186772073569507,-0.163425564373319,
-0.155579823557629,-0.15073619345339,-0.145686377983342,-0.108957740119569,
-0.0721606235587895,-0.0360477125188044,0.),.UNSPECIFIED.);
#6124=B_SPLINE_CURVE_WITH_KNOTS('',3,(#37552,#37553,#37554,#37555,#37556,
#37557,#37558,#37559,#37560,#37561,#37562,#37563,#37564,#37565,#37566,#37567,
#37568,#37569,#37570,#37571,#37572,#37573,#37574,#37575,#37576,#37577,#37578,
#37579,#37580,#37581,#37582,#37583,#37584,#37585,#37586,#37587,#37588,#37589,
#37590,#37591,#37592,#37593,#37594,#37595,#37596,#37597,#37598,#37599,#37600,
#37601,#37602,#37603,#37604,#37605,#37606,#37607,#37608,#37609,#37610,#37611,
#37612,#37613,#37614,#37615,#37616,#37617,#37618,#37619,#37620,#37621,#37622,
#37623,#37624,#37625,#37626,#37627,#37628,#37629,#37630,#37631,#37632,#37633,
#37634,#37635,#37636,#37637,#37638,#37639,#37640,#37641,#37642,#37643,#37644,
#37645,#37646,#37647,#37648),.UNSPECIFIED.,.F.,.F.,(4,3,3,3,3,3,3,3,3,3,
3,3,3,3,3,3,3,3,3,3,3,3,3,3,3,3,3,3,3,3,3,3,4),(-0.741270768406444,-0.707014008746377,
-0.670388059051889,-0.649568879284289,-0.641049525894248,-0.635068301219589,
-0.597844911413426,-0.565274445333034,-0.551024866422862,-0.542258222203151,
-0.537238417066858,-0.501842280952796,-0.466685322391887,-0.432561860623243,
-0.408741691160004,-0.399271293306569,-0.394872553388672,-0.361244518471948,
-0.337281182770287,-0.302985270379873,-0.268599115564268,-0.261938858357407,
-0.257215965685261,-0.223801404360543,-0.190343263618923,-0.157286202950517,
-0.137625427581702,-0.128383055216145,-0.123812703710246,-0.0916026903308386,
-0.0598378393002095,-0.0290475787521256,0.),.UNSPECIFIED.);
#6125=B_SPLINE_CURVE_WITH_KNOTS('',3,(#37905,#37906,#37907,#37908),
 .UNSPECIFIED.,.F.,.F.,(4,4),(57.6587129755276,58.142083558517),
 .UNSPECIFIED.);
#6126=B_SPLINE_CURVE_WITH_KNOTS('',3,(#37910,#37911,#37912,#37913,#37914,
#37915,#37916,#37917,#37918,#37919,#37920,#37921,#37922,#37923,#37924,#37925,
#37926,#37927,#37928,#37929,#37930,#37931,#37932,#37933,#37934,#37935,#37936,
#37937,#37938,#37939,#37940,#37941,#37942,#37943,#37944,#37945,#37946,#37947,
#37948,#37949,#37950,#37951,#37952,#37953,#37954,#37955,#37956,#37957,#37958,
#37959,#37960,#37961,#37962,#37963,#37964,#37965,#37966,#37967,#37968,#37969,
#37970,#37971,#37972,#37973,#37974,#37975,#37976,#37977,#37978,#37979,#37980,
#37981,#37982,#37983,#37984,#37985,#37986,#37987,#37988,#37989,#37990,#37991,
#37992,#37993,#37994,#37995,#37996,#37997,#37998,#37999,#38000,#38001,#38002,
#38003,#38004,#38005,#38006),.UNSPECIFIED.,.F.,.F.,(4,3,3,3,3,3,3,3,3,3,
3,3,3,3,3,3,3,3,3,3,3,3,3,3,3,3,3,3,3,3,3,3,4),(-0.744397949170611,-0.715830617420419,
-0.684607520785607,-0.66522578453741,-0.659137478993546,-0.653541760046644,
-0.621561531951959,-0.59067880805977,-0.576678114100325,-0.571091693875746,
-0.537836424408794,-0.504009574985985,-0.470157175969216,-0.446242817180524,
-0.439103398439934,-0.432971303885224,-0.398062506635795,-0.374499740814447,
-0.340715801391881,-0.306315566008677,-0.298239138263934,-0.292491696861189,
-0.258101090438267,-0.222604447663952,-0.186771987988499,-0.163425489489936,
-0.155579680387924,-0.150736029870234,-0.145686340478701,-0.108957693422131,
-0.0721605833636332,-0.0360477121925127,0.),.UNSPECIFIED.);
#6127=B_SPLINE_CURVE_WITH_KNOTS('',3,(#38007,#38008,#38009,#38010,#38011,
#38012,#38013,#38014,#38015),.UNSPECIFIED.,.F.,.F.,(4,1,1,1,1,1,4),(10.3759343473738,
11.2755500526137,12.2624891535323,13.2494282544508,14.2363673553694,15.223306456288,
15.7079632679489),.UNSPECIFIED.);
#6128=B_SPLINE_CURVE_WITH_KNOTS('',3,(#38019,#38020,#38021,#38022,#38023,
#38024,#38025,#38026),.UNSPECIFIED.,.F.,.F.,(4,1,1,1,1,4),(11.6152142277547,
12.6021533286733,13.5890924295918,14.5760315305104,15.562970631429,15.7079632679489),
 .UNSPECIFIED.);
#6129=B_SPLINE_CURVE_WITH_KNOTS('',3,(#38283,#38284,#38285,#38286,#38287,
#38288,#38289,#38290,#38291,#38292,#38293,#38294,#38295,#38296,#38297,#38298,
#38299,#38300,#38301,#38302,#38303,#38304,#38305,#38306,#38307,#38308,#38309,
#38310,#38311,#38312,#38313,#38314,#38315,#38316,#38317,#38318,#38319,#38320,
#38321,#38322,#38323,#38324,#38325,#38326,#38327,#38328,#38329,#38330,#38331,
#38332,#38333,#38334,#38335,#38336,#38337,#38338,#38339,#38340,#38341,#38342,
#38343,#38344,#38345,#38346,#38347,#38348,#38349,#38350,#38351,#38352,#38353,
#38354,#38355,#38356,#38357,#38358,#38359,#38360,#38361,#38362,#38363,#38364,
#38365,#38366,#38367,#38368,#38369,#38370,#38371,#38372,#38373,#38374,#38375,
#38376,#38377,#38378,#38379),.UNSPECIFIED.,.F.,.F.,(4,3,3,3,3,3,3,3,3,3,
3,3,3,3,3,3,3,3,3,3,3,3,3,3,3,3,3,3,3,3,3,3,4),(-0.741270768406357,-0.707014008746274,
-0.670388059544822,-0.649568879746411,-0.641049544639479,-0.635068332322656,
-0.597844938628606,-0.565274469146312,-0.551024888747808,-0.542258278765346,
-0.537238527650124,-0.501842393489449,-0.466685446597756,-0.432562017839177,
-0.408741809071946,-0.399271703402815,-0.394873316318385,-0.3612453002017,
-0.337281182770253,-0.302985287215554,-0.268599125561966,-0.261938743205762,
-0.25721588929756,-0.22380133845036,-0.190343187133,-0.157286094955077,
-0.137625333085692,-0.128382691599488,-0.123812193525018,-0.091602157735499,
-0.0598372732219336,-0.0290469650055772,0.),.UNSPECIFIED.);
#7607=VERTEX_POINT('',#36737);
#7608=VERTEX_POINT('',#36738);
#7609=VERTEX_POINT('',#36740);
#7610=VERTEX_POINT('',#36751);
#7611=VERTEX_POINT('',#36761);
#7612=VERTEX_POINT('',#36762);
#7613=VERTEX_POINT('',#36809);
#7614=VERTEX_POINT('',#36810);
#7615=VERTEX_POINT('',#36857);
#7616=VERTEX_POINT('',#36858);
#7617=VERTEX_POINT('',#36911);
#7618=VERTEX_POINT('',#36912);
#7619=VERTEX_POINT('',#36959);
#7620=VERTEX_POINT('',#36960);
#7621=VERTEX_POINT('',#37007);
#7622=VERTEX_POINT('',#37008);
#7623=VERTEX_POINT('',#37061);
#7624=VERTEX_POINT('',#37062);
#7625=VERTEX_POINT('',#37109);
#7626=VERTEX_POINT('',#37110);
#7627=VERTEX_POINT('',#37163);
#7628=VERTEX_POINT('',#37164);
#7629=VERTEX_POINT('',#37166);
#7630=VERTEX_POINT('',#37210);
#7631=VERTEX_POINT('',#37211);
#7632=VERTEX_POINT('',#37213);
#7633=VERTEX_POINT('',#37221);
#7634=VERTEX_POINT('',#37230);
#7635=VERTEX_POINT('',#37231);
#7636=VERTEX_POINT('',#37255);
#7637=VERTEX_POINT('',#37256);
#7638=VERTEX_POINT('',#37280);
#7639=VERTEX_POINT('',#37281);
#7640=VERTEX_POINT('',#37305);
#7641=VERTEX_POINT('',#37306);
#7642=VERTEX_POINT('',#37330);
#7643=VERTEX_POINT('',#37331);
#7644=VERTEX_POINT('',#37354);
#7645=VERTEX_POINT('',#37355);
#7646=VERTEX_POINT('',#37379);
#7647=VERTEX_POINT('',#37380);
#7648=VERTEX_POINT('',#37404);
#7649=VERTEX_POINT('',#37405);
#7650=VERTEX_POINT('',#37428);
#7651=VERTEX_POINT('',#37429);
#7652=VERTEX_POINT('',#37432);
#7653=VERTEX_POINT('',#37434);
#7654=VERTEX_POINT('',#37438);
#7655=VERTEX_POINT('',#37440);
#7656=VERTEX_POINT('',#37444);
#7657=VERTEX_POINT('',#37448);
#7658=VERTEX_POINT('',#37550);
#7659=VERTEX_POINT('',#37909);
#7660=VERTEX_POINT('',#38017);
#7661=VERTEX_POINT('',#38383);
#7662=VERTEX_POINT('',#38388);
#9727=EDGE_CURVE('',#7607,#7608,#4515,.T.);
#9728=EDGE_CURVE('',#7607,#7609,#6085,.T.);
#9729=EDGE_CURVE('',#7609,#7610,#1180,.F.);
#9730=EDGE_CURVE('',#7610,#7608,#6086,.T.);
#9731=EDGE_CURVE('',#7611,#7612,#4516,.T.);
#9732=EDGE_CURVE('',#7611,#7607,#6087,.T.);
#9733=EDGE_CURVE('',#7608,#7612,#6088,.T.);
#9734=EDGE_CURVE('',#7613,#7614,#4517,.T.);
#9735=EDGE_CURVE('',#7613,#7611,#6089,.T.);
#9736=EDGE_CURVE('',#7612,#7614,#6090,.T.);
#9737=EDGE_CURVE('',#7615,#7616,#4518,.T.);
#9738=EDGE_CURVE('',#7615,#7613,#6091,.T.);
#9739=EDGE_CURVE('',#7614,#7616,#6092,.T.);
#9740=EDGE_CURVE('',#7617,#7618,#4519,.T.);
#9741=EDGE_CURVE('',#7617,#7615,#6093,.T.);
#9742=EDGE_CURVE('',#7616,#7618,#6094,.T.);
#9743=EDGE_CURVE('',#7619,#7620,#4520,.T.);
#9744=EDGE_CURVE('',#7619,#7617,#6095,.T.);
#9745=EDGE_CURVE('',#7618,#7620,#6096,.T.);
#9746=EDGE_CURVE('',#7621,#7622,#4521,.T.);
#9747=EDGE_CURVE('',#7621,#7619,#6097,.T.);
#9748=EDGE_CURVE('',#7620,#7622,#6098,.T.);
#9749=EDGE_CURVE('',#7623,#7624,#4522,.T.);
#9750=EDGE_CURVE('',#7623,#7621,#6099,.T.);
#9751=EDGE_CURVE('',#7622,#7624,#6100,.T.);
#9752=EDGE_CURVE('',#7625,#7626,#4523,.T.);
#9753=EDGE_CURVE('',#7625,#7623,#6101,.T.);
#9754=EDGE_CURVE('',#7624,#7626,#6102,.T.);
#9755=EDGE_CURVE('',#7627,#7628,#4524,.T.);
#9756=EDGE_CURVE('',#7629,#7627,#1181,.F.);
#9757=EDGE_CURVE('',#7629,#7625,#6103,.T.);
#9758=EDGE_CURVE('',#7626,#7628,#6104,.T.);
#9759=EDGE_CURVE('',#7630,#7631,#4525,.T.);
#9760=EDGE_CURVE('',#7630,#7632,#6105,.T.);
#9761=EDGE_CURVE('',#7633,#7632,#1182,.T.);
#9762=EDGE_CURVE('',#7631,#7633,#6106,.T.);
#9763=EDGE_CURVE('',#7634,#7635,#4526,.T.);
#9764=EDGE_CURVE('',#7634,#7630,#6107,.T.);
#9765=EDGE_CURVE('',#7635,#7631,#6108,.T.);
#9766=EDGE_CURVE('',#7636,#7637,#4527,.T.);
#9767=EDGE_CURVE('',#7636,#7634,#6109,.T.);
#9768=EDGE_CURVE('',#7637,#7635,#6110,.T.);
#9769=EDGE_CURVE('',#7638,#7639,#4528,.T.);
#9770=EDGE_CURVE('',#7638,#7636,#6111,.T.);
#9771=EDGE_CURVE('',#7639,#7637,#6112,.T.);
#9772=EDGE_CURVE('',#7640,#7641,#4529,.T.);
#9773=EDGE_CURVE('',#7640,#7638,#6113,.T.);
#9774=EDGE_CURVE('',#7641,#7639,#6114,.T.);
#9775=EDGE_CURVE('',#7642,#7643,#4530,.T.);
#9776=EDGE_CURVE('',#7642,#7640,#6115,.T.);
#9777=EDGE_CURVE('',#7643,#7641,#6116,.T.);
#9778=EDGE_CURVE('',#7644,#7645,#4531,.T.);
#9779=EDGE_CURVE('',#7644,#7642,#6117,.T.);
#9780=EDGE_CURVE('',#7645,#7643,#6118,.T.);
#9781=EDGE_CURVE('',#7646,#7647,#4532,.T.);
#9782=EDGE_CURVE('',#7646,#7644,#6119,.T.);
#9783=EDGE_CURVE('',#7647,#7645,#6120,.T.);
#9784=EDGE_CURVE('',#7648,#7649,#4533,.T.);
#9785=EDGE_CURVE('',#7648,#7646,#6121,.T.);
#9786=EDGE_CURVE('',#7649,#7647,#6122,.T.);
#9787=EDGE_CURVE('',#7650,#7651,#1183,.T.);
#9788=EDGE_CURVE('',#7651,#7650,#1184,.T.);
#9789=EDGE_CURVE('',#7650,#7652,#4534,.T.);
#9790=EDGE_CURVE('',#7652,#7653,#1185,.T.);
#9791=EDGE_CURVE('',#7653,#7652,#1186,.T.);
#9792=EDGE_CURVE('',#7653,#7654,#4535,.T.);
#9793=EDGE_CURVE('',#7655,#7654,#1187,.T.);
#9794=EDGE_CURVE('',#7654,#7655,#1188,.T.);
#9795=EDGE_CURVE('',#7656,#7656,#1189,.T.);
#9796=EDGE_CURVE('',#7656,#7651,#4536,.T.);
#9797=EDGE_CURVE('',#7655,#7657,#4537,.T.);
#9798=EDGE_CURVE('',#7657,#7657,#1190,.T.);
#9799=EDGE_CURVE('',#7632,#7629,#6123,.T.);
#9800=EDGE_CURVE('',#7658,#7629,#1191,.F.);
#9801=EDGE_CURVE('',#7658,#7633,#6124,.T.);
#9802=EDGE_CURVE('',#7628,#7658,#6125,.T.);
#9803=EDGE_CURVE('',#7659,#7610,#6126,.T.);
#9804=EDGE_CURVE('',#7659,#7649,#6127,.T.);
#9805=EDGE_CURVE('',#7660,#7659,#1192,.T.);
#9806=EDGE_CURVE('',#7660,#7648,#6128,.T.);
#9807=EDGE_CURVE('',#7609,#7660,#6129,.T.);
#9808=EDGE_CURVE('',#7627,#7658,#1193,.F.);
#9809=EDGE_CURVE('',#7661,#7661,#1194,.T.);
#9810=EDGE_CURVE('',#7661,#7656,#4538,.T.);
#9811=EDGE_CURVE('',#7662,#7662,#1195,.T.);
#9812=EDGE_CURVE('',#7662,#7627,#4539,.T.);
#13640=ORIENTED_EDGE('',*,*,#9727,.F.);
#13641=ORIENTED_EDGE('',*,*,#9728,.T.);
#13642=ORIENTED_EDGE('',*,*,#9729,.T.);
#13643=ORIENTED_EDGE('',*,*,#9730,.T.);
#13644=ORIENTED_EDGE('',*,*,#9731,.F.);
#13645=ORIENTED_EDGE('',*,*,#9732,.T.);
#13646=ORIENTED_EDGE('',*,*,#9727,.T.);
#13647=ORIENTED_EDGE('',*,*,#9733,.T.);
#13648=ORIENTED_EDGE('',*,*,#9734,.F.);
#13649=ORIENTED_EDGE('',*,*,#9735,.T.);
#13650=ORIENTED_EDGE('',*,*,#9731,.T.);
#13651=ORIENTED_EDGE('',*,*,#9736,.T.);
#13652=ORIENTED_EDGE('',*,*,#9737,.F.);
#13653=ORIENTED_EDGE('',*,*,#9738,.T.);
#13654=ORIENTED_EDGE('',*,*,#9734,.T.);
#13655=ORIENTED_EDGE('',*,*,#9739,.T.);
#13656=ORIENTED_EDGE('',*,*,#9740,.F.);
#13657=ORIENTED_EDGE('',*,*,#9741,.T.);
#13658=ORIENTED_EDGE('',*,*,#9737,.T.);
#13659=ORIENTED_EDGE('',*,*,#9742,.T.);
#13660=ORIENTED_EDGE('',*,*,#9743,.F.);
#13661=ORIENTED_EDGE('',*,*,#9744,.T.);
#13662=ORIENTED_EDGE('',*,*,#9740,.T.);
#13663=ORIENTED_EDGE('',*,*,#9745,.T.);
#13664=ORIENTED_EDGE('',*,*,#9746,.F.);
#13665=ORIENTED_EDGE('',*,*,#9747,.T.);
#13666=ORIENTED_EDGE('',*,*,#9743,.T.);
#13667=ORIENTED_EDGE('',*,*,#9748,.T.);
#13668=ORIENTED_EDGE('',*,*,#9749,.F.);
#13669=ORIENTED_EDGE('',*,*,#9750,.T.);
#13670=ORIENTED_EDGE('',*,*,#9746,.T.);
#13671=ORIENTED_EDGE('',*,*,#9751,.T.);
#13672=ORIENTED_EDGE('',*,*,#9752,.F.);
#13673=ORIENTED_EDGE('',*,*,#9753,.T.);
#13674=ORIENTED_EDGE('',*,*,#9749,.T.);
#13675=ORIENTED_EDGE('',*,*,#9754,.T.);
#13676=ORIENTED_EDGE('',*,*,#9755,.F.);
#13677=ORIENTED_EDGE('',*,*,#9756,.F.);
#13678=ORIENTED_EDGE('',*,*,#9757,.T.);
#13679=ORIENTED_EDGE('',*,*,#9752,.T.);
#13680=ORIENTED_EDGE('',*,*,#9758,.T.);
#13681=ORIENTED_EDGE('',*,*,#9759,.F.);
#13682=ORIENTED_EDGE('',*,*,#9760,.T.);
#13683=ORIENTED_EDGE('',*,*,#9761,.F.);
#13684=ORIENTED_EDGE('',*,*,#9762,.F.);
#13685=ORIENTED_EDGE('',*,*,#9763,.F.);
#13686=ORIENTED_EDGE('',*,*,#9764,.T.);
#13687=ORIENTED_EDGE('',*,*,#9759,.T.);
#13688=ORIENTED_EDGE('',*,*,#9765,.F.);
#13689=ORIENTED_EDGE('',*,*,#9766,.F.);
#13690=ORIENTED_EDGE('',*,*,#9767,.T.);
#13691=ORIENTED_EDGE('',*,*,#9763,.T.);
#13692=ORIENTED_EDGE('',*,*,#9768,.F.);
#13693=ORIENTED_EDGE('',*,*,#9769,.F.);
#13694=ORIENTED_EDGE('',*,*,#9770,.T.);
#13695=ORIENTED_EDGE('',*,*,#9766,.T.);
#13696=ORIENTED_EDGE('',*,*,#9771,.F.);
#13697=ORIENTED_EDGE('',*,*,#9772,.F.);
#13698=ORIENTED_EDGE('',*,*,#9773,.T.);
#13699=ORIENTED_EDGE('',*,*,#9769,.T.);
#13700=ORIENTED_EDGE('',*,*,#9774,.F.);
#13701=ORIENTED_EDGE('',*,*,#9775,.F.);
#13702=ORIENTED_EDGE('',*,*,#9776,.T.);
#13703=ORIENTED_EDGE('',*,*,#9772,.T.);
#13704=ORIENTED_EDGE('',*,*,#9777,.F.);
#13705=ORIENTED_EDGE('',*,*,#9778,.F.);
#13706=ORIENTED_EDGE('',*,*,#9779,.T.);
#13707=ORIENTED_EDGE('',*,*,#9775,.T.);
#13708=ORIENTED_EDGE('',*,*,#9780,.F.);
#13709=ORIENTED_EDGE('',*,*,#9781,.F.);
#13710=ORIENTED_EDGE('',*,*,#9782,.T.);
#13711=ORIENTED_EDGE('',*,*,#9778,.T.);
#13712=ORIENTED_EDGE('',*,*,#9783,.F.);
#13713=ORIENTED_EDGE('',*,*,#9784,.F.);
#13714=ORIENTED_EDGE('',*,*,#9785,.T.);
#13715=ORIENTED_EDGE('',*,*,#9781,.T.);
#13716=ORIENTED_EDGE('',*,*,#9786,.F.);
#13717=ORIENTED_EDGE('',*,*,#9787,.T.);
#13718=ORIENTED_EDGE('',*,*,#9788,.T.);
#13719=ORIENTED_EDGE('',*,*,#9789,.T.);
#13720=ORIENTED_EDGE('',*,*,#9790,.T.);
#13721=ORIENTED_EDGE('',*,*,#9791,.T.);
#13722=ORIENTED_EDGE('',*,*,#9789,.F.);
#13723=ORIENTED_EDGE('',*,*,#9790,.F.);
#13724=ORIENTED_EDGE('',*,*,#9791,.F.);
#13725=ORIENTED_EDGE('',*,*,#9792,.T.);
#13726=ORIENTED_EDGE('',*,*,#9793,.F.);
#13727=ORIENTED_EDGE('',*,*,#9794,.F.);
#13728=ORIENTED_EDGE('',*,*,#9792,.F.);
#13729=ORIENTED_EDGE('',*,*,#9795,.F.);
#13730=ORIENTED_EDGE('',*,*,#9796,.T.);
#13731=ORIENTED_EDGE('',*,*,#9787,.F.);
#13732=ORIENTED_EDGE('',*,*,#9788,.F.);
#13733=ORIENTED_EDGE('',*,*,#9796,.F.);
#13734=ORIENTED_EDGE('',*,*,#9793,.T.);
#13735=ORIENTED_EDGE('',*,*,#9794,.T.);
#13736=ORIENTED_EDGE('',*,*,#9797,.T.);
#13737=ORIENTED_EDGE('',*,*,#9798,.T.);
#13738=ORIENTED_EDGE('',*,*,#9797,.F.);
#13739=ORIENTED_EDGE('',*,*,#9798,.F.);
#13740=ORIENTED_EDGE('',*,*,#9761,.T.);
#13741=ORIENTED_EDGE('',*,*,#9799,.T.);
#13742=ORIENTED_EDGE('',*,*,#9800,.F.);
#13743=ORIENTED_EDGE('',*,*,#9801,.T.);
#13744=ORIENTED_EDGE('',*,*,#9801,.F.);
#13745=ORIENTED_EDGE('',*,*,#9802,.F.);
#13746=ORIENTED_EDGE('',*,*,#9758,.F.);
#13747=ORIENTED_EDGE('',*,*,#9754,.F.);
#13748=ORIENTED_EDGE('',*,*,#9751,.F.);
#13749=ORIENTED_EDGE('',*,*,#9748,.F.);
#13750=ORIENTED_EDGE('',*,*,#9745,.F.);
#13751=ORIENTED_EDGE('',*,*,#9742,.F.);
#13752=ORIENTED_EDGE('',*,*,#9739,.F.);
#13753=ORIENTED_EDGE('',*,*,#9736,.F.);
#13754=ORIENTED_EDGE('',*,*,#9733,.F.);
#13755=ORIENTED_EDGE('',*,*,#9730,.F.);
#13756=ORIENTED_EDGE('',*,*,#9803,.F.);
#13757=ORIENTED_EDGE('',*,*,#9804,.T.);
#13758=ORIENTED_EDGE('',*,*,#9786,.T.);
#13759=ORIENTED_EDGE('',*,*,#9783,.T.);
#13760=ORIENTED_EDGE('',*,*,#9780,.T.);
#13761=ORIENTED_EDGE('',*,*,#9777,.T.);
#13762=ORIENTED_EDGE('',*,*,#9774,.T.);
#13763=ORIENTED_EDGE('',*,*,#9771,.T.);
#13764=ORIENTED_EDGE('',*,*,#9768,.T.);
#13765=ORIENTED_EDGE('',*,*,#9765,.T.);
#13766=ORIENTED_EDGE('',*,*,#9762,.T.);
#13767=ORIENTED_EDGE('',*,*,#9784,.T.);
#13768=ORIENTED_EDGE('',*,*,#9804,.F.);
#13769=ORIENTED_EDGE('',*,*,#9805,.F.);
#13770=ORIENTED_EDGE('',*,*,#9806,.T.);
#13771=ORIENTED_EDGE('',*,*,#9799,.F.);
#13772=ORIENTED_EDGE('',*,*,#9760,.F.);
#13773=ORIENTED_EDGE('',*,*,#9764,.F.);
#13774=ORIENTED_EDGE('',*,*,#9767,.F.);
#13775=ORIENTED_EDGE('',*,*,#9770,.F.);
#13776=ORIENTED_EDGE('',*,*,#9773,.F.);
#13777=ORIENTED_EDGE('',*,*,#9776,.F.);
#13778=ORIENTED_EDGE('',*,*,#9779,.F.);
#13779=ORIENTED_EDGE('',*,*,#9782,.F.);
#13780=ORIENTED_EDGE('',*,*,#9785,.F.);
#13781=ORIENTED_EDGE('',*,*,#9806,.F.);
#13782=ORIENTED_EDGE('',*,*,#9807,.F.);
#13783=ORIENTED_EDGE('',*,*,#9728,.F.);
#13784=ORIENTED_EDGE('',*,*,#9732,.F.);
#13785=ORIENTED_EDGE('',*,*,#9735,.F.);
#13786=ORIENTED_EDGE('',*,*,#9738,.F.);
#13787=ORIENTED_EDGE('',*,*,#9741,.F.);
#13788=ORIENTED_EDGE('',*,*,#9744,.F.);
#13789=ORIENTED_EDGE('',*,*,#9747,.F.);
#13790=ORIENTED_EDGE('',*,*,#9750,.F.);
#13791=ORIENTED_EDGE('',*,*,#9753,.F.);
#13792=ORIENTED_EDGE('',*,*,#9757,.F.);
#13793=ORIENTED_EDGE('',*,*,#9755,.T.);
#13794=ORIENTED_EDGE('',*,*,#9802,.T.);
#13795=ORIENTED_EDGE('',*,*,#9808,.F.);
#13796=ORIENTED_EDGE('',*,*,#9809,.F.);
#13797=ORIENTED_EDGE('',*,*,#9810,.T.);
#13798=ORIENTED_EDGE('',*,*,#9795,.T.);
#13799=ORIENTED_EDGE('',*,*,#9810,.F.);
#13800=ORIENTED_EDGE('',*,*,#9809,.T.);
#13801=ORIENTED_EDGE('',*,*,#9807,.T.);
#13802=ORIENTED_EDGE('',*,*,#9805,.T.);
#13803=ORIENTED_EDGE('',*,*,#9803,.T.);
#13804=ORIENTED_EDGE('',*,*,#9729,.F.);
#13805=ORIENTED_EDGE('',*,*,#9811,.F.);
#13806=ORIENTED_EDGE('',*,*,#9812,.T.);
#13807=ORIENTED_EDGE('',*,*,#9808,.T.);
#13808=ORIENTED_EDGE('',*,*,#9800,.T.);
#13809=ORIENTED_EDGE('',*,*,#9756,.T.);
#13810=ORIENTED_EDGE('',*,*,#9812,.F.);
#13811=ORIENTED_EDGE('',*,*,#9811,.T.);
#15932=PLANE('',#18362);
#15933=PLANE('',#18363);
#15934=PLANE('',#18371);
#15935=PLANE('',#18374);
#16583=ADVANCED_FACE('',(#2412),#1470,.T.);
#16584=ADVANCED_FACE('',(#2413),#1471,.T.);
#16585=ADVANCED_FACE('',(#2414),#1472,.T.);
#16586=ADVANCED_FACE('',(#2415),#1473,.T.);
#16587=ADVANCED_FACE('',(#2416),#1474,.T.);
#16588=ADVANCED_FACE('',(#2417),#1475,.T.);
#16589=ADVANCED_FACE('',(#2418),#1476,.T.);
#16590=ADVANCED_FACE('',(#2419),#1477,.T.);
#16591=ADVANCED_FACE('',(#2420),#1478,.T.);
#16592=ADVANCED_FACE('',(#2421),#1479,.T.);
#16593=ADVANCED_FACE('',(#2422),#1480,.T.);
#16594=ADVANCED_FACE('',(#2423),#1481,.T.);
#16595=ADVANCED_FACE('',(#2424),#1482,.T.);
#16596=ADVANCED_FACE('',(#2425),#1483,.T.);
#16597=ADVANCED_FACE('',(#2426),#1484,.T.);
#16598=ADVANCED_FACE('',(#2427),#1485,.T.);
#16599=ADVANCED_FACE('',(#2428),#1486,.T.);
#16600=ADVANCED_FACE('',(#2429),#1487,.T.);
#16601=ADVANCED_FACE('',(#2430),#1488,.T.);
#16602=ADVANCED_FACE('',(#2431),#643,.T.);
#16603=ADVANCED_FACE('',(#2432),#644,.T.);
#16604=ADVANCED_FACE('',(#2433),#1489,.T.);
#16605=ADVANCED_FACE('',(#2434),#645,.T.);
#16606=ADVANCED_FACE('',(#2435),#15932,.T.);
#16607=ADVANCED_FACE('',(#2436),#15933,.F.);
#16608=ADVANCED_FACE('',(#2437),#355,.F.);
#16609=ADVANCED_FACE('',(#2438),#1490,.T.);
#16610=ADVANCED_FACE('',(#2439),#356,.F.);
#16611=ADVANCED_FACE('',(#2440),#1491,.T.);
#16612=ADVANCED_FACE('',(#2441),#646,.T.);
#16613=ADVANCED_FACE('',(#2442,#559),#15934,.T.);
#16614=ADVANCED_FACE('',(#2443),#647,.T.);
#16615=ADVANCED_FACE('',(#2444),#15935,.T.);
#16965=CLOSED_SHELL('',(#16583,#16584,#16585,#16586,#16587,#16588,#16589,
#16590,#16591,#16592,#16593,#16594,#16595,#16596,#16597,#16598,#16599,#16600,
#16601,#16602,#16603,#16604,#16605,#16606,#16607,#16608,#16609,#16610,#16611,
#16612,#16613,#16614,#16615));
#18327=AXIS2_PLACEMENT_3D('',#36735,#21677,#21678);
#18328=AXIS2_PLACEMENT_3D('',#36736,#21679,#21680);
#18329=AXIS2_PLACEMENT_3D('',#36752,#21682,#21683);
#18330=AXIS2_PLACEMENT_3D('',#36760,#21684,#21685);
#18331=AXIS2_PLACEMENT_3D('',#36808,#21687,#21688);
#18332=AXIS2_PLACEMENT_3D('',#36856,#21690,#21691);
#18333=AXIS2_PLACEMENT_3D('',#36910,#21693,#21694);
#18334=AXIS2_PLACEMENT_3D('',#36958,#21696,#21697);
#18335=AXIS2_PLACEMENT_3D('',#37006,#21699,#21700);
#18336=AXIS2_PLACEMENT_3D('',#37060,#21702,#21703);
#18337=AXIS2_PLACEMENT_3D('',#37108,#21705,#21706);
#18338=AXIS2_PLACEMENT_3D('',#37162,#21708,#21709);
#18339=AXIS2_PLACEMENT_3D('',#37167,#21711,#21712);
#18340=AXIS2_PLACEMENT_3D('',#37209,#21713,#21714);
#18341=AXIS2_PLACEMENT_3D('',#37222,#21716,#21717);
#18342=AXIS2_PLACEMENT_3D('',#37229,#21718,#21719);
#18343=AXIS2_PLACEMENT_3D('',#37254,#21721,#21722);
#18344=AXIS2_PLACEMENT_3D('',#37279,#21724,#21725);
#18345=AXIS2_PLACEMENT_3D('',#37304,#21727,#21728);
#18346=AXIS2_PLACEMENT_3D('',#37329,#21730,#21731);
#18347=AXIS2_PLACEMENT_3D('',#37353,#21733,#21734);
#18348=AXIS2_PLACEMENT_3D('',#37378,#21736,#21737);
#18349=AXIS2_PLACEMENT_3D('',#37403,#21739,#21740);
#18350=AXIS2_PLACEMENT_3D('',#37427,#21742,#21743);
#18351=AXIS2_PLACEMENT_3D('',#37430,#21744,#21745);
#18352=AXIS2_PLACEMENT_3D('',#37431,#21746,#21747);
#18353=AXIS2_PLACEMENT_3D('',#37435,#21749,#21750);
#18354=AXIS2_PLACEMENT_3D('',#37436,#21751,#21752);
#18355=AXIS2_PLACEMENT_3D('',#37437,#21753,#21754);
#18356=AXIS2_PLACEMENT_3D('',#37441,#21756,#21757);
#18357=AXIS2_PLACEMENT_3D('',#37442,#21758,#21759);
#18358=AXIS2_PLACEMENT_3D('',#37443,#21760,#21761);
#18359=AXIS2_PLACEMENT_3D('',#37445,#21762,#21763);
#18360=AXIS2_PLACEMENT_3D('',#37447,#21765,#21766);
#18361=AXIS2_PLACEMENT_3D('',#37450,#21768,#21769);
#18362=AXIS2_PLACEMENT_3D('',#37451,#21770,#21771);
#18363=AXIS2_PLACEMENT_3D('',#37452,#21772,#21773);
#18364=AXIS2_PLACEMENT_3D('',#37551,#21774,#21775);
#18365=AXIS2_PLACEMENT_3D('',#38016,#21776,#21777);
#18366=AXIS2_PLACEMENT_3D('',#38018,#21778,#21779);
#18367=AXIS2_PLACEMENT_3D('',#38380,#21780,#21781);
#18368=AXIS2_PLACEMENT_3D('',#38381,#21782,#21783);
#18369=AXIS2_PLACEMENT_3D('',#38382,#21784,#21785);
#18370=AXIS2_PLACEMENT_3D('',#38384,#21786,#21787);
#18371=AXIS2_PLACEMENT_3D('',#38386,#21789,#21790);
#18372=AXIS2_PLACEMENT_3D('',#38387,#21791,#21792);
#18373=AXIS2_PLACEMENT_3D('',#38389,#21793,#21794);
#18374=AXIS2_PLACEMENT_3D('',#38391,#21796,#21797);
#21677=DIRECTION('axis',(0.,0.,1.));
#21678=DIRECTION('refdir',(1.,0.,0.));
#21679=DIRECTION('center_axis',(1.,0.,0.));
#21680=DIRECTION('ref_axis',(0.,1.,0.));
#21681=DIRECTION('',(-1.,0.,0.));
#21682=DIRECTION('center_axis',(-1.,0.,0.));
#21683=DIRECTION('ref_axis',(0.,1.,0.));
#21684=DIRECTION('center_axis',(1.,0.,0.));
#21685=DIRECTION('ref_axis',(0.,1.,0.));
#21686=DIRECTION('',(-1.,0.,0.));
#21687=DIRECTION('center_axis',(1.,0.,0.));
#21688=DIRECTION('ref_axis',(0.,1.,0.));
#21689=DIRECTION('',(-1.,0.,0.));
#21690=DIRECTION('center_axis',(1.,0.,0.));
#21691=DIRECTION('ref_axis',(0.,1.,0.));
#21692=DIRECTION('',(-1.,0.,0.));
#21693=DIRECTION('center_axis',(1.,0.,0.));
#21694=DIRECTION('ref_axis',(0.,1.,0.));
#21695=DIRECTION('',(-1.,0.,0.));
#21696=DIRECTION('center_axis',(1.,0.,0.));
#21697=DIRECTION('ref_axis',(0.,1.,0.));
#21698=DIRECTION('',(-1.,0.,0.));
#21699=DIRECTION('center_axis',(1.,0.,0.));
#21700=DIRECTION('ref_axis',(0.,1.,0.));
#21701=DIRECTION('',(-1.,0.,0.));
#21702=DIRECTION('center_axis',(1.,0.,0.));
#21703=DIRECTION('ref_axis',(0.,1.,0.));
#21704=DIRECTION('',(-1.,0.,0.));
#21705=DIRECTION('center_axis',(1.,0.,0.));
#21706=DIRECTION('ref_axis',(0.,1.,0.));
#21707=DIRECTION('',(-1.,0.,0.));
#21708=DIRECTION('center_axis',(1.,0.,0.));
#21709=DIRECTION('ref_axis',(0.,1.,0.));
#21710=DIRECTION('',(-1.,0.,0.));
#21711=DIRECTION('center_axis',(-1.,0.,0.));
#21712=DIRECTION('ref_axis',(0.,1.,0.));
#21713=DIRECTION('center_axis',(1.,0.,0.));
#21714=DIRECTION('ref_axis',(0.,0.315640347057222,-0.948878902341915));
#21715=DIRECTION('',(1.,0.,0.));
#21716=DIRECTION('center_axis',(1.,0.,0.));
#21717=DIRECTION('ref_axis',(0.,1.,5.66627894982857E-14));
#21718=DIRECTION('center_axis',(1.,0.,0.));
#21719=DIRECTION('ref_axis',(0.,1.,5.66627894982857E-14));
#21720=DIRECTION('',(1.,0.,0.));
#21721=DIRECTION('center_axis',(1.,0.,0.));
#21722=DIRECTION('ref_axis',(0.,1.,5.66627894982857E-14));
#21723=DIRECTION('',(1.,0.,0.));
#21724=DIRECTION('center_axis',(1.,0.,0.));
#21725=DIRECTION('ref_axis',(0.,1.,5.66627894982857E-14));
#21726=DIRECTION('',(1.,0.,0.));
#21727=DIRECTION('center_axis',(1.,0.,0.));
#21728=DIRECTION('ref_axis',(0.,1.,5.66627894982857E-14));
#21729=DIRECTION('',(1.,0.,0.));
#21730=DIRECTION('center_axis',(1.,0.,0.));
#21731=DIRECTION('ref_axis',(0.,1.,5.66627894982857E-14));
#21732=DIRECTION('',(1.,0.,0.));
#21733=DIRECTION('center_axis',(1.,0.,0.));
#21734=DIRECTION('ref_axis',(0.,1.,5.66627894982857E-14));
#21735=DIRECTION('',(1.,0.,0.));
#21736=DIRECTION('center_axis',(1.,0.,0.));
#21737=DIRECTION('ref_axis',(0.,1.,5.66627894982857E-14));
#21738=DIRECTION('',(1.,0.,0.));
#21739=DIRECTION('center_axis',(1.,0.,0.));
#21740=DIRECTION('ref_axis',(0.,1.,5.66627894982857E-14));
#21741=DIRECTION('',(1.,0.,0.));
#21742=DIRECTION('center_axis',(1.,0.,6.92018220157537E-16));
#21743=DIRECTION('ref_axis',(0.,-1.,-3.00652077147108E-17));
#21744=DIRECTION('center_axis',(-1.,0.,0.));
#21745=DIRECTION('ref_axis',(0.,-1.,0.));
#21746=DIRECTION('center_axis',(-1.,0.,0.));
#21747=DIRECTION('ref_axis',(0.,-1.,0.));
#21748=DIRECTION('',(-0.923879532511287,-0.382683432365088,-6.97712130664736E-16));
#21749=DIRECTION('center_axis',(1.,0.,0.));
#21750=DIRECTION('ref_axis',(0.,-1.,-6.12323399573677E-17));
#21751=DIRECTION('center_axis',(1.,0.,0.));
#21752=DIRECTION('ref_axis',(0.,-1.,-6.12323399573677E-17));
#21753=DIRECTION('center_axis',(1.,0.,0.));
#21754=DIRECTION('ref_axis',(0.,1.,0.));
#21755=DIRECTION('',(-0.707106781186548,0.707106781186547,8.65956056235493E-17));
#21756=DIRECTION('center_axis',(-1.,0.,0.));
#21757=DIRECTION('ref_axis',(0.,-1.,-6.12323399573677E-17));
#21758=DIRECTION('center_axis',(-1.,0.,0.));
#21759=DIRECTION('ref_axis',(0.,-1.,-6.12323399573677E-17));
#21760=DIRECTION('center_axis',(1.,0.,0.));
#21761=DIRECTION('ref_axis',(0.,1.,0.));
#21762=DIRECTION('center_axis',(1.,0.,0.));
#21763=DIRECTION('ref_axis',(0.,0.,-1.));
#21764=DIRECTION('',(-1.,0.,0.));
#21765=DIRECTION('center_axis',(1.,0.,-1.61995324118126E-15));
#21766=DIRECTION('ref_axis',(0.,-1.,-3.20798861992349E-17));
#21767=DIRECTION('',(-0.382683432365089,-0.923879532511287,4.7714870511266E-16));
#21768=DIRECTION('center_axis',(1.,0.,0.));
#21769=DIRECTION('ref_axis',(0.,-1.,0.));
#21770=DIRECTION('center_axis',(-1.,0.,0.));
#21771=DIRECTION('ref_axis',(0.,0.,1.));
#21772=DIRECTION('center_axis',(1.,0.,0.));
#21773=DIRECTION('ref_axis',(0.,0.,-1.));
#21774=DIRECTION('center_axis',(-1.,0.,0.));
#21775=DIRECTION('ref_axis',(0.,1.,0.));
#21776=DIRECTION('center_axis',(1.,0.,0.));
#21777=DIRECTION('ref_axis',(0.,1.,5.66627894982857E-14));
#21778=DIRECTION('center_axis',(-1.,0.,0.));
#21779=DIRECTION('ref_axis',(0.,1.,5.66627894982857E-14));
#21780=DIRECTION('center_axis',(1.,0.,0.));
#21781=DIRECTION('ref_axis',(0.,-0.970927363150326,-0.23937429996964));
#21782=DIRECTION('center_axis',(-1.,0.,0.));
#21783=DIRECTION('ref_axis',(0.,1.,0.));
#21784=DIRECTION('center_axis',(-1.,0.,0.));
#21785=DIRECTION('ref_axis',(0.,1.,0.));
#21786=DIRECTION('center_axis',(1.,0.,0.));
#21787=DIRECTION('ref_axis',(0.,0.,-1.));
#21788=DIRECTION('',(-0.707106781186547,-0.707106781186548,-8.65956056235493E-17));
#21789=DIRECTION('center_axis',(1.,0.,0.));
#21790=DIRECTION('ref_axis',(0.,0.,-1.));
#21791=DIRECTION('center_axis',(-1.,0.,0.));
#21792=DIRECTION('ref_axis',(0.,1.,0.));
#21793=DIRECTION('center_axis',(1.,0.,0.));
#21794=DIRECTION('ref_axis',(0.,0.,-1.));
#21795=DIRECTION('',(-0.707106781186546,-0.707106781186549,-8.65956056235495E-17));
#21796=DIRECTION('center_axis',(1.,0.,0.));
#21797=DIRECTION('ref_axis',(0.,0.,-1.));
#36735=CARTESIAN_POINT('',(0.,0.,0.));
#36736=CARTESIAN_POINT('Origin',(23.75,0.,0.));
#36737=CARTESIAN_POINT('',(18.404163522035,-3.93613844682217,0.0030445838845216));
#36738=CARTESIAN_POINT('',(18.220836477965,-3.93627057114866,0.00387085077091485));
#36739=CARTESIAN_POINT('',(23.75,-3.933,-4.81653586104654E-16));
#36740=CARTESIAN_POINT('',(18.,1.74869447533107,3.5228619944509));
#36741=CARTESIAN_POINT('Ctrl Pts',(18.404163522035,-3.93613844682217,0.0030445838845216));
#36742=CARTESIAN_POINT('Ctrl Pts',(18.3945483991958,-3.93767917958426,0.192676392097596));
#36743=CARTESIAN_POINT('Ctrl Pts',(18.3849332763566,-3.92513522773623,0.38209457511149));
#36744=CARTESIAN_POINT('Ctrl Pts',(18.3753181535174,-3.89779650413505,0.569340254555103));
#36745=CARTESIAN_POINT('Ctrl Pts',(18.3098697216666,-3.71170667268696,1.84388830717668));
#36746=CARTESIAN_POINT('Ctrl Pts',(18.2444212898158,-2.84013321415606,3.01777812376358));
#36747=CARTESIAN_POINT('Ctrl Pts',(18.178972857965,-1.67389089476471,3.56551633596367));
#36748=CARTESIAN_POINT('Ctrl Pts',(18.1193152386434,-0.610836542511951,
4.06479121279916));
#36749=CARTESIAN_POINT('Ctrl Pts',(18.0596576193217,0.697049477382223,4.04381518476905));
#36750=CARTESIAN_POINT('Ctrl Pts',(18.,1.75280451302835,3.52727163111204));
#36751=CARTESIAN_POINT('',(18.,-1.74869447533112,3.52286199445088));
#36752=CARTESIAN_POINT('Origin',(18.,0.,0.));
#36753=CARTESIAN_POINT('Ctrl Pts',(18.,-1.74869447533111,3.52286199445088));
#36754=CARTESIAN_POINT('Ctrl Pts',(18.0654484318508,-2.90764455848562,2.94757701002937));
#36755=CARTESIAN_POINT('Ctrl Pts',(18.1308968637015,-3.7512349686817,1.76098836716689));
#36756=CARTESIAN_POINT('Ctrl Pts',(18.1963452955523,-3.90885202961768,0.484525031295026));
#36757=CARTESIAN_POINT('Ctrl Pts',(18.2045090230232,-3.92851243543427,0.325305039219235));
#36758=CARTESIAN_POINT('Ctrl Pts',(18.2126727504941,-3.93749985993302,0.164686697017349));
#36759=CARTESIAN_POINT('Ctrl Pts',(18.220836477965,-3.93627057114866,0.00387085077091485));
#36760=CARTESIAN_POINT('Origin',(23.75,0.,0.));
#36761=CARTESIAN_POINT('',(19.654163522035,-3.92689321902701,-0.000266995866781417));
#36762=CARTESIAN_POINT('',(19.470836477965,-3.9268765274925,0.000201000649742641));
#36763=CARTESIAN_POINT('',(23.75,-3.933,-4.81653586104654E-16));
#36764=CARTESIAN_POINT('Ctrl Pts',(19.654163522035,-3.92689321902701,-0.000266995866781417));
#36765=CARTESIAN_POINT('Ctrl Pts',(19.6205723236338,-3.92647671847103,0.666255959009758));
#36766=CARTESIAN_POINT('Ctrl Pts',(19.5869811252325,-3.76529862270708,1.33296720638558));
#36767=CARTESIAN_POINT('Ctrl Pts',(19.5533899268313,-3.44451966305658,1.91112423318315));
#36768=CARTESIAN_POINT('Ctrl Pts',(19.4879414949806,-2.81952023228035,3.03759403981093));
#36769=CARTESIAN_POINT('Ctrl Pts',(19.4224930631298,-1.58864622066021,3.82789554528875));
#36770=CARTESIAN_POINT('Ctrl Pts',(19.357044631279,-0.304251272167243,3.92740159534381));
#36771=CARTESIAN_POINT('Ctrl Pts',(19.2915961994282,0.980143676325715,4.02690764539886));
#36772=CARTESIAN_POINT('Ctrl Pts',(19.2261477675775,2.3180595616915,3.43561824003117));
#36773=CARTESIAN_POINT('Ctrl Pts',(19.1606993357267,3.10909064786165,2.41883077544061));
#36774=CARTESIAN_POINT('Ctrl Pts',(19.0952509038759,3.9001217340318,1.40204331085005));
#36775=CARTESIAN_POINT('Ctrl Pts',(19.0298024720251,4.14426802100631,-0.0402422129633744));
#36776=CARTESIAN_POINT('Ctrl Pts',(18.9643540401743,3.7319893739621,-1.26070538200933));
#36777=CARTESIAN_POINT('Ctrl Pts',(18.8989056083236,3.31971072691789,-2.48116855105527));
#36778=CARTESIAN_POINT('Ctrl Pts',(18.8334571764728,2.25100714585497,-3.47980936533375));
#36779=CARTESIAN_POINT('Ctrl Pts',(18.768008744622,1.00542163713921,-3.80865813843412));
#36780=CARTESIAN_POINT('Ctrl Pts',(18.7025603127713,-0.240163871576541,
-4.13750691153448));
#36781=CARTESIAN_POINT('Ctrl Pts',(18.6371118809205,-1.66263130794512,-3.79656364345673));
#36782=CARTESIAN_POINT('Ctrl Pts',(18.5716634490697,-2.62356192394677,-2.93848886508973));
#36783=CARTESIAN_POINT('Ctrl Pts',(18.5158301400581,-3.44332084718932,-2.20647508109503));
#36784=CARTESIAN_POINT('Ctrl Pts',(18.4599968310465,-3.92719168557441,-1.09811361486684));
#36785=CARTESIAN_POINT('Ctrl Pts',(18.404163522035,-3.93613844682217,0.0030445838845216));
#36786=CARTESIAN_POINT('Ctrl Pts',(18.220836477965,-3.93627057114866,0.00387085077091485));
#36787=CARTESIAN_POINT('Ctrl Pts',(18.2781211823449,-3.92764467754057,-1.12457056825791));
#36788=CARTESIAN_POINT('Ctrl Pts',(18.3354058867248,-3.41596831095298,-2.26273669035632));
#36789=CARTESIAN_POINT('Ctrl Pts',(18.3926905911047,-2.55888297838309,-2.99573282302492));
#36790=CARTESIAN_POINT('Ctrl Pts',(18.4581390229554,-1.57965315453669,-3.83318931259173));
#36791=CARTESIAN_POINT('Ctrl Pts',(18.5235874548062,-0.149549795168021,
-4.14176426284409));
#36792=CARTESIAN_POINT('Ctrl Pts',(18.589035886657,1.08866631561176,-3.78545010096408));
#36793=CARTESIAN_POINT('Ctrl Pts',(18.6544843185077,2.32688242639155,-3.42913593908406));
#36794=CARTESIAN_POINT('Ctrl Pts',(18.7199327503585,3.37321128858245,-2.40793266507167));
#36795=CARTESIAN_POINT('Ctrl Pts',(18.7853811822093,3.75861745519042,-1.1788821270789));
#36796=CARTESIAN_POINT('Ctrl Pts',(18.8508296140601,4.14402362179839,0.0501684109138591));
#36797=CARTESIAN_POINT('Ctrl Pts',(18.9162780459109,3.86850709282343,1.48706621288699));
#36798=CARTESIAN_POINT('Ctrl Pts',(18.9817264777616,3.05544614190684,2.48637190452309));
#36799=CARTESIAN_POINT('Ctrl Pts',(19.0471749096124,2.24238519099026,3.4856775961592));
#36800=CARTESIAN_POINT('Ctrl Pts',(19.1126233414632,0.891779818132044,4.04739117745827));
#36801=CARTESIAN_POINT('Ctrl Pts',(19.178071773314,-0.390146913530757,3.91976270565962));
#36802=CARTESIAN_POINT('Ctrl Pts',(19.2435202051647,-1.67207364519356,3.79213423386097));
#36803=CARTESIAN_POINT('Ctrl Pts',(19.3089686370155,-2.88532173566096,2.97516370896458));
#36804=CARTESIAN_POINT('Ctrl Pts',(19.3744170688663,-3.48551032220533,1.83530485432315));
#36805=CARTESIAN_POINT('Ctrl Pts',(19.4065568718992,-3.78024531292475,1.27555364199425));
#36806=CARTESIAN_POINT('Ctrl Pts',(19.4386966749321,-3.92714077791773,0.637937789729678));
#36807=CARTESIAN_POINT('Ctrl Pts',(19.470836477965,-3.9268765274925,0.000201000649742641));
#36808=CARTESIAN_POINT('Origin',(23.75,0.,0.));
#36809=CARTESIAN_POINT('',(20.904163522035,-3.93705835258154,-0.00244415858371427));
#36810=CARTESIAN_POINT('',(20.720836477965,-3.93634147379978,-0.00275764000347982));
#36811=CARTESIAN_POINT('',(23.75,-3.933,-4.81653586104654E-16));
#36812=CARTESIAN_POINT('Ctrl Pts',(20.904163522035,-3.93705835258154,-0.00244415858371427));
#36813=CARTESIAN_POINT('Ctrl Pts',(20.8465962480717,-3.92872844902641,1.13228879098002));
#36814=CARTESIAN_POINT('Ctrl Pts',(20.7890289741085,-3.41049682016329,2.27366756012711));
#36815=CARTESIAN_POINT('Ctrl Pts',(20.7314617001453,-2.54581885219839,3.00597915976938));
#36816=CARTESIAN_POINT('Ctrl Pts',(20.6660132682945,-1.5627634951674,3.83854673719779));
#36817=CARTESIAN_POINT('Ctrl Pts',(20.6005648364438,-0.131909118660247,
4.14237477626342));
#36818=CARTESIAN_POINT('Ctrl Pts',(20.535116404593,1.10464315307146,3.78111974646024));
#36819=CARTESIAN_POINT('Ctrl Pts',(20.4696679727422,2.34119542480316,3.41986471665706));
#36820=CARTESIAN_POINT('Ctrl Pts',(20.4042195408914,3.38344559175942,2.39352661798506));
#36821=CARTESIAN_POINT('Ctrl Pts',(20.3387711090406,3.76367980962101,1.1626776497403));
#36822=CARTESIAN_POINT('Ctrl Pts',(20.2733226771899,4.14391402748261,-0.0681713185044673));
#36823=CARTESIAN_POINT('Ctrl Pts',(20.2078742453391,3.86213229624954,-1.503531156322));
#36824=CARTESIAN_POINT('Ctrl Pts',(20.1424258134883,3.04478561004353,-2.49927715158322));
#36825=CARTESIAN_POINT('Ctrl Pts',(20.0769773816376,2.22743892383752,-3.49502314684444));
#36826=CARTESIAN_POINT('Ctrl Pts',(20.0115289497868,0.874527282658571,-4.05115529954934));
#36827=CARTESIAN_POINT('Ctrl Pts',(19.946080517936,-0.40682594379375,-3.9181104320261));
#36828=CARTESIAN_POINT('Ctrl Pts',(19.8806320860852,-1.68817917024607,-3.78506556450286));
#36829=CARTESIAN_POINT('Ctrl Pts',(19.8151836542344,-2.89797398197177,-2.96284367675147));
#36830=CARTESIAN_POINT('Ctrl Pts',(19.7497352223837,-3.49330896286845,-1.82041367898691));
#36831=CARTESIAN_POINT('Ctrl Pts',(19.7178779889341,-3.78309016817464,-1.2643322250943));
#36832=CARTESIAN_POINT('Ctrl Pts',(19.6860207554845,-3.92728821998187,-0.632384288003329));
#36833=CARTESIAN_POINT('Ctrl Pts',(19.654163522035,-3.92689321902701,-0.000266995866781417));
#36834=CARTESIAN_POINT('Ctrl Pts',(19.470836477965,-3.9268765274925,0.000201000649742641));
#36835=CARTESIAN_POINT('Ctrl Pts',(19.5041451067829,-3.92660266709205,-0.66072831398253));
#36836=CARTESIAN_POINT('Ctrl Pts',(19.5374537356008,-3.76827097225227,-1.32178752157556));
#36837=CARTESIAN_POINT('Ctrl Pts',(19.5707623644186,-3.45263815106435,-1.89643882110259));
#36838=CARTESIAN_POINT('Ctrl Pts',(19.6362107962694,-2.83244831075765,-3.02557645750042));
#36839=CARTESIAN_POINT('Ctrl Pts',(19.7016592281202,-1.60493954752288,-3.8211045459096));
#36840=CARTESIAN_POINT('Ctrl Pts',(19.7671076599709,-0.320979108461926,
-3.92607034958216));
#36841=CARTESIAN_POINT('Ctrl Pts',(19.8325560918217,0.962981330599031,-4.03103615325472));
#36842=CARTESIAN_POINT('Ctrl Pts',(19.8980045236725,2.30339344548619,-3.44543967219065));
#36843=CARTESIAN_POINT('Ctrl Pts',(19.9634529555233,3.09875161344691,-2.43204719578226));
#36844=CARTESIAN_POINT('Ctrl Pts',(20.028901387374,3.89410978140763,-1.41865471937386));
#36845=CARTESIAN_POINT('Ctrl Pts',(20.0943498192248,4.14441400244192,0.022533752378857));
#36846=CARTESIAN_POINT('Ctrl Pts',(20.1597982510756,3.73733454864532,1.24476807205102));
#36847=CARTESIAN_POINT('Ctrl Pts',(20.2252466829264,3.33025509484873,2.46700239172319));
#36848=CARTESIAN_POINT('Ctrl Pts',(20.2906951147771,2.26579196622125,3.4702825593148));
#36849=CARTESIAN_POINT('Ctrl Pts',(20.3561435466279,1.02162940702816,3.80438874667093));
#36850=CARTESIAN_POINT('Ctrl Pts',(20.4215919784787,-0.222533152164935,
4.13849493402707));
#36851=CARTESIAN_POINT('Ctrl Pts',(20.4870404103295,-1.64639514192364,3.80342714114774));
#36852=CARTESIAN_POINT('Ctrl Pts',(20.5524888421803,-2.61099445316008,2.94954526738738));
#36853=CARTESIAN_POINT('Ctrl Pts',(20.6086047207752,-3.4380476966283,2.21742181985246));
#36854=CARTESIAN_POINT('Ctrl Pts',(20.6647205993701,-3.92747625062555,1.1038947635718));
#36855=CARTESIAN_POINT('Ctrl Pts',(20.720836477965,-3.93634147379978,-0.00275764000347982));
#36856=CARTESIAN_POINT('Origin',(23.75,0.,0.));
#36857=CARTESIAN_POINT('',(22.154163522035,-3.93253297961002,0.00339845520594975));
#36858=CARTESIAN_POINT('',(21.970836477965,-3.93336915469688,0.00337969667030601));
#36859=CARTESIAN_POINT('',(23.75,-3.933,-4.81653586104654E-16));
#36860=CARTESIAN_POINT('Ctrl Pts',(22.154163522035,-3.93253297961002,0.00339845520594975));
#36861=CARTESIAN_POINT('Ctrl Pts',(22.1380686043605,-3.93532255328355,0.32159861761589));
#36862=CARTESIAN_POINT('Ctrl Pts',(22.1219736866861,-3.89986016195786,0.639185244649252));
#36863=CARTESIAN_POINT('Ctrl Pts',(22.1058787690116,-3.82372336883648,0.94670144792028));
#36864=CARTESIAN_POINT('Ctrl Pts',(22.0404303371608,-3.51412043598972,2.19718645690713));
#36865=CARTESIAN_POINT('Ctrl Pts',(21.97498190531,-2.5319402955714,3.2811505782075));
#36866=CARTESIAN_POINT('Ctrl Pts',(21.9095334734592,-1.31793994286403,3.71216087310869));
#36867=CARTESIAN_POINT('Ctrl Pts',(21.8440850416085,-0.103939590156664,
4.14317116800988));
#36868=CARTESIAN_POINT('Ctrl Pts',(21.7786366097577,1.34188097483974,3.92122763651189));
#36869=CARTESIAN_POINT('Ctrl Pts',(21.7131881779069,2.3707043932351,3.14592827253841));
#36870=CARTESIAN_POINT('Ctrl Pts',(21.6477397460562,3.39952781163046,2.37062890856494));
#36871=CARTESIAN_POINT('Ctrl Pts',(21.5822913142054,4.01135408342477,1.04197371211599));
#36872=CARTESIAN_POINT('Ctrl Pts',(21.5168428823546,3.93162388784021,-0.24379836679225));
#36873=CARTESIAN_POINT('Ctrl Pts',(21.4513944505038,3.85189369225565,-1.52957044570049));
#36874=CARTESIAN_POINT('Ctrl Pts',(21.3859460186531,3.08060702929222,-2.77245940706802));
#36875=CARTESIAN_POINT('Ctrl Pts',(21.3204975868023,1.96388166738833,-3.41471417252903));
#36876=CARTESIAN_POINT('Ctrl Pts',(21.2550491549515,0.84715630548443,-4.05696893799003));
#36877=CARTESIAN_POINT('Ctrl Pts',(21.1896007231007,-0.615007755359946,
-4.09858950754451));
#36878=CARTESIAN_POINT('Ctrl Pts',(21.1241522912499,-1.76645896380458,-3.52089855434547));
#36879=CARTESIAN_POINT('Ctrl Pts',(21.0587038593992,-2.91791017224922,-2.94320760114644));
#36880=CARTESIAN_POINT('Ctrl Pts',(20.9932554275484,-3.75864852829412,-1.74620512519392));
#36881=CARTESIAN_POINT('Ctrl Pts',(20.9278069956976,-3.91138953753916,-0.467050329322068));
#36882=CARTESIAN_POINT('Ctrl Pts',(20.9199258378101,-3.92978227783443,-0.313017289510358));
#36883=CARTESIAN_POINT('Ctrl Pts',(20.9120446799225,-3.93819874504042,-0.157793003857012));
#36884=CARTESIAN_POINT('Ctrl Pts',(20.904163522035,-3.93705835258154,-0.00244415858371427));
#36885=CARTESIAN_POINT('Ctrl Pts',(20.720836477965,-3.93634147379978,-0.00275764000347982));
#36886=CARTESIAN_POINT('Ctrl Pts',(20.7301690312209,-3.93781583666231,-0.186803452894212));
#36887=CARTESIAN_POINT('Ctrl Pts',(20.7395015844767,-3.92599851426311,-0.370659122854381));
#36888=CARTESIAN_POINT('Ctrl Pts',(20.7488341377326,-3.90023200959619,-0.552538626230935));
#36889=CARTESIAN_POINT('Ctrl Pts',(20.8142825695833,-3.71953362208168,-1.8280446914475));
#36890=CARTESIAN_POINT('Ctrl Pts',(20.8797310014341,-2.8528002143385,-3.00636086723926));
#36891=CARTESIAN_POINT('Ctrl Pts',(20.9451794332849,-1.68898196160953,-3.55871417944791));
#36892=CARTESIAN_POINT('Ctrl Pts',(21.0106278651357,-0.525163708880573,
-4.11106749165656));
#36893=CARTESIAN_POINT('Ctrl Pts',(21.0760762969865,0.935739388834165,-4.0374579402821));
#36894=CARTESIAN_POINT('Ctrl Pts',(21.1415247288372,2.03814179849579,-3.37091767673898));
#36895=CARTESIAN_POINT('Ctrl Pts',(21.206973160688,3.14054420815743,-2.70437741319586));
#36896=CARTESIAN_POINT('Ctrl Pts',(21.2724215925388,3.88444592976595,-1.44490643748405));
#36897=CARTESIAN_POINT('Ctrl Pts',(21.3378700243896,3.936018208958,-0.157697248386007));
#36898=CARTESIAN_POINT('Ctrl Pts',(21.4033184562403,3.98759048815004,1.12951194071202));
#36899=CARTESIAN_POINT('Ctrl Pts',(21.4687668880911,3.34683332492562,2.44445934319629));
#36900=CARTESIAN_POINT('Ctrl Pts',(21.5342153199419,2.30128892652022,3.19705752490842));
#36901=CARTESIAN_POINT('Ctrl Pts',(21.5996637517926,1.25574452811482,3.94965570662055));
#36902=CARTESIAN_POINT('Ctrl Pts',(21.6651121836434,-0.194587105471541,
4.13990466756053));
#36903=CARTESIAN_POINT('Ctrl Pts',(21.7305606154942,-1.3988642776945,3.68242942294792));
#36904=CARTESIAN_POINT('Ctrl Pts',(21.796009047345,-2.60314144991746,3.22495417833531));
#36905=CARTESIAN_POINT('Ctrl Pts',(21.8614574791958,-3.561364160777,2.11975472817009));
#36906=CARTESIAN_POINT('Ctrl Pts',(21.9269059110465,-3.84352638982112,0.862793468370925));
#36907=CARTESIAN_POINT('Ctrl Pts',(21.9415494333527,-3.90665775566324,0.581559224473073));
#36908=CARTESIAN_POINT('Ctrl Pts',(21.9561929556589,-3.93594539582555,0.292727753415705));
#36909=CARTESIAN_POINT('Ctrl Pts',(21.970836477965,-3.93336915469688,0.00337969667030601));
#36910=CARTESIAN_POINT('Origin',(23.75,0.,0.));
#36911=CARTESIAN_POINT('',(23.404163522035,-3.92812465671341,-0.00212229078741105));
#36912=CARTESIAN_POINT('',(23.220836477965,-3.92768863108871,-0.00174943043258178));
#36913=CARTESIAN_POINT('',(23.75,-3.933,-4.81653586104654E-16));
#36914=CARTESIAN_POINT('Ctrl Pts',(23.404163522035,-3.92812465671341,-0.00212229078741105));
#36915=CARTESIAN_POINT('Ctrl Pts',(23.3640925287985,-3.92414083826686,0.792347133215219));
#36916=CARTESIAN_POINT('Ctrl Pts',(23.324021535562,-3.68976240124988,1.58897831133289));
#36917=CARTESIAN_POINT('Ctrl Pts',(23.2839505423256,-3.24164538944974,2.23804361037454));
#36918=CARTESIAN_POINT('Ctrl Pts',(23.2185021104748,-2.5097305218822,3.29816971556831));
#36919=CARTESIAN_POINT('Ctrl Pts',(23.153053678624,-1.20762356863968,3.96463315855812));
#36920=CARTESIAN_POINT('Ctrl Pts',(23.0876052467732,0.0803501277369667,
3.93835598823379));
#36921=CARTESIAN_POINT('Ctrl Pts',(23.0221568149224,1.3683238241136,3.91207881790945));
#36922=CARTESIAN_POINT('Ctrl Pts',(22.9567083830717,2.64216426362435,3.19306103427099));
#36923=CARTESIAN_POINT('Ctrl Pts',(22.8912599512209,3.33023080703671,2.10396454450698));
#36924=CARTESIAN_POINT('Ctrl Pts',(22.8258115193701,4.01829735044907,1.01486805474297));
#36925=CARTESIAN_POINT('Ctrl Pts',(22.7603630875193,4.12058999776305,-0.444307141146586));
#36926=CARTESIAN_POINT('Ctrl Pts',(22.6949146556685,3.59120454263221,-1.61875074232297));
#36927=CARTESIAN_POINT('Ctrl Pts',(22.6294662238178,3.06181908750136,-2.79319434349935));
#36928=CARTESIAN_POINT('Ctrl Pts',(22.564017791967,1.90075552992569,-3.68290634996255));
#36929=CARTESIAN_POINT('Ctrl Pts',(22.4985693601163,0.62904546370725,-3.88862518619208));
#36930=CARTESIAN_POINT('Ctrl Pts',(22.4331209282655,-0.642664602511191,
-4.0943440224216));
#36931=CARTESIAN_POINT('Ctrl Pts',(22.3676724964147,-2.02502117737241,-3.61606968841744));
#36932=CARTESIAN_POINT('Ctrl Pts',(22.3022240645639,-2.89768660216542,-2.66842957307869));
#36933=CARTESIAN_POINT('Ctrl Pts',(22.2528705503876,-3.55574828822536,-1.95383078829727));
#36934=CARTESIAN_POINT('Ctrl Pts',(22.2035170362113,-3.92397902073757,-0.972331681725521));
#36935=CARTESIAN_POINT('Ctrl Pts',(22.154163522035,-3.93253297961002,0.00339845520594975));
#36936=CARTESIAN_POINT('Ctrl Pts',(21.970836477965,-3.93336915469688,0.00337969667030601));
#36937=CARTESIAN_POINT('Ctrl Pts',(22.0216413875096,-3.92443102527893,-1.00049775456773));
#36938=CARTESIAN_POINT('Ctrl Pts',(22.0724462970542,-3.53194559205172,-2.01059337634254));
#36939=CARTESIAN_POINT('Ctrl Pts',(22.1232512065988,-2.83859494485778,-2.73120603295504));
#36940=CARTESIAN_POINT('Ctrl Pts',(22.1886996384496,-1.94539952362163,-3.65952120504872));
#36941=CARTESIAN_POINT('Ctrl Pts',(22.2541480703004,-0.55290693392065,-4.10742847980296));
#36942=CARTESIAN_POINT('Ctrl Pts',(22.3195965021512,0.713996594007594,-3.8739277927898));
#36943=CARTESIAN_POINT('Ctrl Pts',(22.385044934002,1.98090012193584,-3.64042710577664));
#36944=CARTESIAN_POINT('Ctrl Pts',(22.4504933658528,3.12221458809134,-2.72551845699607));
#36945=CARTESIAN_POINT('Ctrl Pts',(22.5159417977035,3.62577087549378,-1.53977051229877));
#36946=CARTESIAN_POINT('Ctrl Pts',(22.5813902295543,4.12932716289623,-0.35402256760147));
#36947=CARTESIAN_POINT('Ctrl Pts',(22.646838661405,3.99512527154563,1.10256467301257));
#36948=CARTESIAN_POINT('Ctrl Pts',(22.7122870932558,3.28338880059249,2.17634226495933));
#36949=CARTESIAN_POINT('Ctrl Pts',(22.7777355251066,2.57165232963934,3.25011985690608));
#36950=CARTESIAN_POINT('Ctrl Pts',(22.8431839569574,1.28238127908365,3.94108780018556));
#36951=CARTESIAN_POINT('Ctrl Pts',(22.9086323888082,-0.00585916808317544,
3.93917165702054));
#36952=CARTESIAN_POINT('Ctrl Pts',(22.974080820659,-1.29409961525001,3.93725551385553));
#36953=CARTESIAN_POINT('Ctrl Pts',(23.0395292525097,-2.58130945902797,3.24245528424603));
#36954=CARTESIAN_POINT('Ctrl Pts',(23.1049776843605,-3.28984849000153,2.16656515823267));
#36955=CARTESIAN_POINT('Ctrl Pts',(23.1435972822287,-3.7079408976622,1.53170741081231));
#36956=CARTESIAN_POINT('Ctrl Pts',(23.1822168800969,-3.92454558560357,0.764157755427278));
#36957=CARTESIAN_POINT('Ctrl Pts',(23.220836477965,-3.92768863108871,-0.00174943043258178));
#36958=CARTESIAN_POINT('Origin',(23.75,0.,0.));
#36959=CARTESIAN_POINT('',(24.654163522035,-3.93909475595853,-0.000490377207084114));
#36960=CARTESIAN_POINT('',(24.470836477965,-3.93885420654145,-0.000985259163277196));
#36961=CARTESIAN_POINT('',(23.75,-3.933,-4.81653586104654E-16));
#36962=CARTESIAN_POINT('Ctrl Pts',(24.654163522035,-3.93909475595853,-0.000490377207084114));
#36963=CARTESIAN_POINT('Ctrl Pts',(24.5901164532365,-3.93683716814358,1.26023770975936));
#36964=CARTESIAN_POINT('Ctrl Pts',(24.526069384438,-3.27732068913603,2.52300066969272));
#36965=CARTESIAN_POINT('Ctrl Pts',(24.4620223156395,-2.24041894240288,3.24000416594111));
#36966=CARTESIAN_POINT('Ctrl Pts',(24.3965738837887,-1.18082957195824,3.9726958463149));
#36967=CARTESIAN_POINT('Ctrl Pts',(24.331125451938,0.272840271641166,4.13548412538781));
#36968=CARTESIAN_POINT('Ctrl Pts',(24.2656770200872,1.46825083487448,3.6553171570425));
#36969=CARTESIAN_POINT('Ctrl Pts',(24.2002285882364,2.6636613981078,3.17515018869718));
#36970=CARTESIAN_POINT('Ctrl Pts',(24.1347801563856,3.60081268097502,2.05202797293364));
#36971=CARTESIAN_POINT('Ctrl Pts',(24.0693317245348,3.85915455648697,0.789955784984271));
#36972=CARTESIAN_POINT('Ctrl Pts',(24.0038832926841,4.11749643199892,-0.472116402965099));
#36973=CARTESIAN_POINT('Ctrl Pts',(23.9384348608333,3.69702890015558,-1.8731385631003));
#36974=CARTESIAN_POINT('Ctrl Pts',(23.8729864289825,2.78643833118525,-2.7843967855499));
#36975=CARTESIAN_POINT('Ctrl Pts',(23.8075379971318,1.87584776221493,-3.6956550079995));
#36976=CARTESIAN_POINT('Ctrl Pts',(23.742089565281,0.475134156117602,-4.11714929276351));
#36977=CARTESIAN_POINT('Ctrl Pts',(23.6766411334302,-0.787127042068175,
-3.85973251049337));
#36978=CARTESIAN_POINT('Ctrl Pts',(23.6111927015794,-2.04938824025396,-3.60231572822324));
#36979=CARTESIAN_POINT('Ctrl Pts',(23.5457442697286,-3.1731970305282,-2.66598787891895));
#36980=CARTESIAN_POINT('Ctrl Pts',(23.4802958378779,-3.65424003471902,-1.47092957056794));
#36981=CARTESIAN_POINT('Ctrl Pts',(23.4549183992636,-3.84076305695926,-1.00754919607961));
#36982=CARTESIAN_POINT('Ctrl Pts',(23.4295409606493,-3.9306476565173,-0.505269265946798));
#36983=CARTESIAN_POINT('Ctrl Pts',(23.404163522035,-3.92812465671341,-0.00212229078741105));
#36984=CARTESIAN_POINT('Ctrl Pts',(23.220836477965,-3.92768863108871,-0.00174943043258178));
#36985=CARTESIAN_POINT('Ctrl Pts',(23.2476653119476,-3.92987208845688,-0.533821173013996));
#36986=CARTESIAN_POINT('Ctrl Pts',(23.2744941459302,-3.8290387712291,-1.06510025837181));
#36987=CARTESIAN_POINT('Ctrl Pts',(23.3013229799128,-3.62117429826454,-1.55054970043114));
#36988=CARTESIAN_POINT('Ctrl Pts',(23.3667714117636,-3.11409285738485,-2.73479441066429));
#36989=CARTESIAN_POINT('Ctrl Pts',(23.4322198436144,-1.97006175745636,-3.64630380871338));
#36990=CARTESIAN_POINT('Ctrl Pts',(23.4976682754651,-0.702469213319956,
-3.87603465885666));
#36991=CARTESIAN_POINT('Ctrl Pts',(23.5631167073159,0.565123330816479,-4.10576550899994));
#36992=CARTESIAN_POINT('Ctrl Pts',(23.6285651391667,1.95627731916084,-3.65371781123739));
#36993=CARTESIAN_POINT('Ctrl Pts',(23.6940135710175,2.8467072206701,-2.72274965281462));
#36994=CARTESIAN_POINT('Ctrl Pts',(23.7594620028682,3.73713712217935,-1.79178149439185));
#36995=CARTESIAN_POINT('Ctrl Pts',(23.824910434719,4.12684293685351,-0.381892875308882));
#36996=CARTESIAN_POINT('Ctrl Pts',(23.8903588665698,3.84094272963275,0.874223438163058));
#36997=CARTESIAN_POINT('Ctrl Pts',(23.9558072984206,3.55504252241199,2.13033975163501));
#36998=CARTESIAN_POINT('Ctrl Pts',(24.0212557302713,2.59353629329628,3.23268375949592));
#36999=CARTESIAN_POINT('Ctrl Pts',(24.0867041621221,1.38790354194334,3.68657448458775));
#37000=CARTESIAN_POINT('Ctrl Pts',(24.1521525939729,0.182270790590404,4.14046520967958));
#37001=CARTESIAN_POINT('Ctrl Pts',(24.2176010258237,-1.26748848299976,3.94590265200234));
#37002=CARTESIAN_POINT('Ctrl Pts',(24.2830494576745,-2.31078940792255,3.19019748359728));
#37003=CARTESIAN_POINT('Ctrl Pts',(24.3456451311047,-3.30861505689732,2.46743190169848));
#37004=CARTESIAN_POINT('Ctrl Pts',(24.4082408045348,-3.93464344142654,1.2313756263831));
#37005=CARTESIAN_POINT('Ctrl Pts',(24.470836477965,-3.93885420654145,-0.000985259163277196));
#37006=CARTESIAN_POINT('Origin',(23.75,0.,0.));
#37007=CARTESIAN_POINT('',(25.904163522035,-3.92919769550165,0.00273228871909281));
#37008=CARTESIAN_POINT('',(25.720836477965,-3.92985825803548,0.00297976440258395));
#37009=CARTESIAN_POINT('',(23.75,-3.933,-4.81653586104654E-16));
#37010=CARTESIAN_POINT('Ctrl Pts',(25.904163522035,-3.92919769550165,0.00273228871909281));
#37011=CARTESIAN_POINT('Ctrl Pts',(25.8815888095252,-3.93213961178236,0.450002964145652));
#37012=CARTESIAN_POINT('Ctrl Pts',(25.8590140970155,-3.8614845501863,0.896372500728469));
#37013=CARTESIAN_POINT('Ctrl Pts',(25.8364393845058,-3.71312585452063,1.31521879246953));
#37014=CARTESIAN_POINT('Ctrl Pts',(25.770990952655,-3.28300547187737,2.52953472092949));
#37015=CARTESIAN_POINT('Ctrl Pts',(25.7055425208042,-2.19976150773091,3.51250908524159));
#37016=CARTESIAN_POINT('Ctrl Pts',(25.6400940889535,-0.949503751846705,
3.82302846763078));
#37017=CARTESIAN_POINT('Ctrl Pts',(25.5746456571027,0.300754004037498,4.13354785001997));
#37018=CARTESIAN_POINT('Ctrl Pts',(25.5091972252519,1.71802555165944,3.77161225048626));
#37019=CARTESIAN_POINT('Ctrl Pts',(25.4437487934011,2.66630502260462,2.89964162311381));
#37020=CARTESIAN_POINT('Ctrl Pts',(25.3783003615503,3.61458449354981,2.02767099574135));
#37021=CARTESIAN_POINT('Ctrl Pts',(25.3128519296996,4.09387188781823,0.645665340530145));
#37022=CARTESIAN_POINT('Ctrl Pts',(25.2474034978488,3.88908519554681,-0.626195163358931));
#37023=CARTESIAN_POINT('Ctrl Pts',(25.181955065998,3.6842985032754,-1.898055667248));
#37024=CARTESIAN_POINT('Ctrl Pts',(25.1165066341473,2.79543772446416,-3.05977101981493));
#37025=CARTESIAN_POINT('Ctrl Pts',(25.0510582022965,1.62138244634291,-3.59001713026159));
#37026=CARTESIAN_POINT('Ctrl Pts',(24.9856097704457,0.447327168221664,-4.12026324070824));
#37027=CARTESIAN_POINT('Ctrl Pts',(24.9201613385949,-1.0119226092096,-4.01904010903461));
#37028=CARTESIAN_POINT('Ctrl Pts',(24.8547129067441,-2.1015231180563,-3.33177199326797));
#37029=CARTESIAN_POINT('Ctrl Pts',(24.7892644748934,-3.191123626903,-2.64450387750133));
#37030=CARTESIAN_POINT('Ctrl Pts',(24.7238160430426,-3.91107486716513,-1.37119077764169));
#37031=CARTESIAN_POINT('Ctrl Pts',(24.6583676111918,-3.93829603865126,-0.0832366868745308));
#37032=CARTESIAN_POINT('Ctrl Pts',(24.6569662481396,-3.93887889056813,-0.0556593832661226));
#37033=CARTESIAN_POINT('Ctrl Pts',(24.6555648850873,-3.93914415244474,-0.0280753673276151));
#37034=CARTESIAN_POINT('Ctrl Pts',(24.654163522035,-3.93909475595853,-0.000490377207084114));
#37035=CARTESIAN_POINT('Ctrl Pts',(24.470836477965,-3.93885420654145,-0.000985259163277196));
#37036=CARTESIAN_POINT('Ctrl Pts',(24.4736892363856,-3.93904610951143,-0.0571493309080139));
#37037=CARTESIAN_POINT('Ctrl Pts',(24.4765419948062,-3.93794648282358,-0.113305727242253));
#37038=CARTESIAN_POINT('Ctrl Pts',(24.4793947532268,-3.9355316597942,-0.16940551076599));
#37039=CARTESIAN_POINT('Ctrl Pts',(24.5448431850775,-3.88013041048765,-1.45645555759133));
#37040=CARTESIAN_POINT('Ctrl Pts',(24.6102916169283,-3.13248533561915,-2.71370787210913));
#37041=CARTESIAN_POINT('Ctrl Pts',(24.6757400487791,-2.02810494588332,-3.37696579793198));
#37042=CARTESIAN_POINT('Ctrl Pts',(24.7411884806299,-0.923724556147519,
-4.04022372375482));
#37043=CARTESIAN_POINT('Ctrl Pts',(24.8066369124807,0.537391148455583,-4.10948726088273));
#37044=CARTESIAN_POINT('Ctrl Pts',(24.8720853443314,1.69956105657403,-3.55367413911433));
#37045=CARTESIAN_POINT('Ctrl Pts',(24.9375337761822,2.8617309646925,-2.99786101734593));
#37046=CARTESIAN_POINT('Ctrl Pts',(25.002982208033,3.7249550763263,-1.81697123668122));
#37047=CARTESIAN_POINT('Ctrl Pts',(25.0684306398838,3.90185835737233,-0.540933482350884));
#37048=CARTESIAN_POINT('Ctrl Pts',(25.1338790717345,4.07876163841836,0.735104271979422));
#37049=CARTESIAN_POINT('Ctrl Pts',(25.1993275035853,3.56934408887662,2.10628999997535));
#37050=CARTESIAN_POINT('Ctrl Pts',(25.2647759354361,2.60220873153787,2.95729900206465));
#37051=CARTESIAN_POINT('Ctrl Pts',(25.3302243672869,1.63507337419909,3.80830800415396));
#37052=CARTESIAN_POINT('Ctrl Pts',(25.3956727991376,0.21022020906327,4.13914028033664));
#37053=CARTESIAN_POINT('Ctrl Pts',(25.4611212309884,-1.0329426038841,3.80133361456278));
#37054=CARTESIAN_POINT('Ctrl Pts',(25.5265696628392,-2.27610541683143,3.46352694878893));
#37055=CARTESIAN_POINT('Ctrl Pts',(25.59201809469,-3.3375778775903,2.45708134105862));
#37056=CARTESIAN_POINT('Ctrl Pts',(25.6574665265407,-3.74102026390006,1.2336430055299));
#37057=CARTESIAN_POINT('Ctrl Pts',(25.6785898436822,-3.87123028167017,0.838781352873692));
#37058=CARTESIAN_POINT('Ctrl Pts',(25.6997131608236,-3.93289597643157,0.421316448174291));
#37059=CARTESIAN_POINT('Ctrl Pts',(25.720836477965,-3.92985825803548,0.00297976440258395));
#37060=CARTESIAN_POINT('Origin',(23.75,0.,0.));
#37061=CARTESIAN_POINT('',(27.154163522035,-3.93098047339281,-0.00325343987953419));
#37062=CARTESIAN_POINT('',(26.970836477965,-3.93023513714109,-0.00309016900265477));
#37063=CARTESIAN_POINT('',(23.75,-3.933,-4.81653586104654E-16));
#37064=CARTESIAN_POINT('Ctrl Pts',(27.154163522035,-3.93098047339281,-0.00325343987953419));
#37065=CARTESIAN_POINT('Ctrl Pts',(27.1076127339632,-3.92351105440917,0.917992942990856));
#37066=CARTESIAN_POINT('Ctrl Pts',(27.0610619458915,-3.59950298381568,1.84397406686046));
#37067=CARTESIAN_POINT('Ctrl Pts',(27.0145111578198,-3.00784466327321,2.54361478474492));
#37068=CARTESIAN_POINT('Ctrl Pts',(26.949062725969,-2.17599818172083,3.52727993288205));
#37069=CARTESIAN_POINT('Ctrl Pts',(26.8836142941182,-0.815083000998221,
4.06353423725179));
#37070=CARTESIAN_POINT('Ctrl Pts',(26.8181658622674,0.464183581722977,3.9117308993607));
#37071=CARTESIAN_POINT('Ctrl Pts',(26.7527174304166,1.74345016444418,3.75992756146961));
#37072=CARTESIAN_POINT('Ctrl Pts',(26.6872689985659,2.94106814916398,2.92006658131768));
#37073=CARTESIAN_POINT('Ctrl Pts',(26.6218205667151,3.51960279979861,1.76903905110911));
#37074=CARTESIAN_POINT('Ctrl Pts',(26.5563721348643,4.09813745043322,0.618011520900572));
#37075=CARTESIAN_POINT('Ctrl Pts',(26.4909237030135,4.0575887669827,-0.84418255936459));
#37076=CARTESIAN_POINT('Ctrl Pts',(26.4254752711628,3.41615271487111,-1.96137833317676));
#37077=CARTESIAN_POINT('Ctrl Pts',(26.360026839312,2.77471666275951,-3.07857410698896));
#37078=CARTESIAN_POINT('Ctrl Pts',(26.2945784074612,1.53239324198682,-3.85077157434815));
#37079=CARTESIAN_POINT('Ctrl Pts',(26.2291299756104,0.246679921490786,-3.93144415461087));
#37080=CARTESIAN_POINT('Ctrl Pts',(26.1636815437597,-1.03903339900524,-4.01211673487358));
#37081=CARTESIAN_POINT('Ctrl Pts',(26.0982331119089,-2.3681366192246,-3.40126442803983));
#37082=CARTESIAN_POINT('Ctrl Pts',(26.0327846800581,-3.14418982876426,-2.37300952831905));
#37083=CARTESIAN_POINT('Ctrl Pts',(25.9899109607171,-3.65256392664006,-1.69942406973689));
#37084=CARTESIAN_POINT('Ctrl Pts',(25.947037241376,-3.92361043086253,-0.84672071757979));
#37085=CARTESIAN_POINT('Ctrl Pts',(25.904163522035,-3.92919769550165,0.00273228871909281));
#37086=CARTESIAN_POINT('Ctrl Pts',(25.720836477965,-3.92985825803548,0.00297976440258395));
#37087=CARTESIAN_POINT('Ctrl Pts',(25.7651615926744,-3.92348391751595,-0.874856863772733));
#37088=CARTESIAN_POINT('Ctrl Pts',(25.8094867073837,-3.63220286020098,-1.75653217218374));
#37089=CARTESIAN_POINT('Ctrl Pts',(25.8538118220931,-3.09150438011423,-2.44125138467072));
#37090=CARTESIAN_POINT('Ctrl Pts',(25.9192602539439,-2.29313379815808,-3.4522763760154));
#37091=CARTESIAN_POINT('Ctrl Pts',(25.9847086857946,-0.950980322385189,
-4.03389529537762));
#37092=CARTESIAN_POINT('Ctrl Pts',(26.0501571176454,0.332659693891018,-3.92510448349789));
#37093=CARTESIAN_POINT('Ctrl Pts',(26.1156055494962,1.61629971016724,-3.81631367161816));
#37094=CARTESIAN_POINT('Ctrl Pts',(26.1810539813469,2.84142626694679,-3.01711312849645));
#37095=CARTESIAN_POINT('Ctrl Pts',(26.2465024131977,3.45825923142778,-1.8861470808627));
#37096=CARTESIAN_POINT('Ctrl Pts',(26.3119508450485,4.07509219590877,-0.755181033228954));
#37097=CARTESIAN_POINT('Ctrl Pts',(26.3773992768993,4.08363156809121,0.707550518916832));
#37098=CARTESIAN_POINT('Ctrl Pts',(26.44284770875,3.48004533087329,1.84564136168573));
#37099=CARTESIAN_POINT('Ctrl Pts',(26.5082961406008,2.87645909365536,2.98373220445462));
#37100=CARTESIAN_POINT('Ctrl Pts',(26.5737445724516,1.66074724703709,3.79718233784663));
#37101=CARTESIAN_POINT('Ctrl Pts',(26.6391930043024,0.378464894959196,3.92095295644834));
#37102=CARTESIAN_POINT('Ctrl Pts',(26.7046414361532,-0.903817457118713,
4.04472357505004));
#37103=CARTESIAN_POINT('Ctrl Pts',(26.7700898680039,-2.25267031465624,3.47881467886142));
#37104=CARTESIAN_POINT('Ctrl Pts',(26.8355382998547,-3.06279071672218,2.4771800499131));
#37105=CARTESIAN_POINT('Ctrl Pts',(26.8806376925581,-3.6210308015747,1.78697079357367));
#37106=CARTESIAN_POINT('Ctrl Pts',(26.9257370852616,-3.92346175853291,0.889863626098021));
#37107=CARTESIAN_POINT('Ctrl Pts',(26.970836477965,-3.93023513714109,-0.00309016900265477));
#37108=CARTESIAN_POINT('Origin',(23.75,0.,0.));
#37109=CARTESIAN_POINT('',(28.404163522035,-3.93818417569795,0.00170700930730246));
#37110=CARTESIAN_POINT('',(28.220836477965,-3.93866152695812,0.00124115044389661));
#37111=CARTESIAN_POINT('',(23.75,-3.933,-4.81653586104654E-16));
#37112=CARTESIAN_POINT('Ctrl Pts',(28.404163522035,-3.93818417569795,0.00170700930730246));
#37113=CARTESIAN_POINT('Ctrl Pts',(28.399085090252,-3.9387267147927,0.101734442167589));
#37114=CARTESIAN_POINT('Ctrl Pts',(28.394006658469,-3.93523450213126,0.201722834433012));
#37115=CARTESIAN_POINT('Ctrl Pts',(28.388928226686,-3.92758354814724,0.301391698975487));
#37116=CARTESIAN_POINT('Ctrl Pts',(28.3234797948353,-3.82898166437366,1.58587698250684));
#37117=CARTESIAN_POINT('Ctrl Pts',(28.2580313629845,-3.03966117892474,2.81729242473998));
#37118=CARTESIAN_POINT('Ctrl Pts',(28.1925829311337,-1.91366888952096,3.44310820754633));
#37119=CARTESIAN_POINT('Ctrl Pts',(28.1271344992829,-0.787676600117176,
4.06892399035268));
#37120=CARTESIAN_POINT('Ctrl Pts',(28.0616860674322,0.674987493241486,4.08914011373224));
#37121=CARTESIAN_POINT('Ctrl Pts',(27.9962376355814,1.81786335315111,3.49464730782801));
#37122=CARTESIAN_POINT('Ctrl Pts',(27.9307892037306,2.96073921306072,2.90015450192379));
#37123=CARTESIAN_POINT('Ctrl Pts',(27.8653407718798,3.7838268395213,1.69095276673577));
#37124=CARTESIAN_POINT('Ctrl Pts',(27.7998923400291,3.91780578128033,0.409694993734216));
#37125=CARTESIAN_POINT('Ctrl Pts',(27.7344439081783,4.05178472303937,-0.871562779267352));
#37126=CARTESIAN_POINT('Ctrl Pts',(27.6689954763275,3.49665498009686,-2.22487659008246));
#37127=CARTESIAN_POINT('Ctrl Pts',(27.6035470444767,2.50151091037662,-3.04295164422803));
#37128=CARTESIAN_POINT('Ctrl Pts',(27.538098612626,1.50636684065638,-3.86102669837359));
#37129=CARTESIAN_POINT('Ctrl Pts',(27.4726501807752,0.0712084441584163,
-4.14386299584961));
#37130=CARTESIAN_POINT('Ctrl Pts',(27.4072017489244,-1.15992021363229,-3.76453165356687));
#37131=CARTESIAN_POINT('Ctrl Pts',(27.3417533170736,-2.39104887142302,-3.38520031128414));
#37132=CARTESIAN_POINT('Ctrl Pts',(27.2763048852229,-3.41814779050649,-2.34370132924263));
#37133=CARTESIAN_POINT('Ctrl Pts',(27.2108564533721,-3.78030835885712,-1.10741384226963));
#37134=CARTESIAN_POINT('Ctrl Pts',(27.191958809593,-3.88487895310921,-0.750446992543413));
#37135=CARTESIAN_POINT('Ctrl Pts',(27.173061165814,-3.93401274040774,-0.377240362493561));
#37136=CARTESIAN_POINT('Ctrl Pts',(27.154163522035,-3.93098047339281,-0.00325343987953419));
#37137=CARTESIAN_POINT('Ctrl Pts',(26.970836477965,-3.93023513714109,-0.00309016900265477));
#37138=CARTESIAN_POINT('Ctrl Pts',(26.9911855171124,-3.9332913145793,-0.405994745850263));
#37139=CARTESIAN_POINT('Ctrl Pts',(27.0115345562597,-3.87615595376113,-0.808053757116241));
#37140=CARTESIAN_POINT('Ctrl Pts',(27.031883595407,-3.75516863334752,-1.18988033548289));
#37141=CARTESIAN_POINT('Ctrl Pts',(27.0973320272578,-3.36603820131256,-2.41794573022264));
#37142=CARTESIAN_POINT('Ctrl Pts',(27.1627804591086,-2.31638939064824,-3.43671615799411));
#37143=CARTESIAN_POINT('Ctrl Pts',(27.2282288909594,-1.07725517871138,-3.789014376074));
#37144=CARTESIAN_POINT('Ctrl Pts',(27.2936773228101,0.161879033225451,-4.14131259415387));
#37145=CARTESIAN_POINT('Ctrl Pts',(27.3591257546609,1.59049864643482,-3.82713860254219));
#37146=CARTESIAN_POINT('Ctrl Pts',(27.4245741865117,2.56750366718156,-2.98747957947988));
#37147=CARTESIAN_POINT('Ctrl Pts',(27.4900226183624,3.54450868792831,-2.14782055641755));
#37148=CARTESIAN_POINT('Ctrl Pts',(27.5554710502132,4.06989911621242,-0.782676501904576));
#37149=CARTESIAN_POINT('Ctrl Pts',(27.620919482064,3.90790720462131,0.49533994505792));
#37150=CARTESIAN_POINT('Ctrl Pts',(27.6863679139148,3.74591529303021,1.7733563920204));
#37151=CARTESIAN_POINT('Ctrl Pts',(27.7518163457656,2.8965410415639,2.9642452314324));
#37152=CARTESIAN_POINT('Ctrl Pts',(27.8172647776163,1.74093814691504,3.53358903245858));
#37153=CARTESIAN_POINT('Ctrl Pts',(27.8827132094671,0.585335252266155,4.10293283348478));
#37154=CARTESIAN_POINT('Ctrl Pts',(27.9481616413179,-0.876496285565295,
4.05073159612515));
#37155=CARTESIAN_POINT('Ctrl Pts',(28.0136100731687,-1.98854212366733,3.40041399637644));
#37156=CARTESIAN_POINT('Ctrl Pts',(28.0790585050194,-3.10058796176937,2.75009639662773));
#37157=CARTESIAN_POINT('Ctrl Pts',(28.1445069368702,-3.862848100142,1.50166243448994));
#37158=CARTESIAN_POINT('Ctrl Pts',(28.209955368721,-3.93327883257213,0.215345311481923));
#37159=CARTESIAN_POINT('Ctrl Pts',(28.2135824051357,-3.93718197927882,0.144059890058629));
#37160=CARTESIAN_POINT('Ctrl Pts',(28.2172094415504,-3.93896039300732,0.0726581226105382));
#37161=CARTESIAN_POINT('Ctrl Pts',(28.220836477965,-3.93866152695812,0.00124115044389661));
#37162=CARTESIAN_POINT('Origin',(23.75,0.,0.));
#37163=CARTESIAN_POINT('',(29.567,-3.933,-4.81653586104654E-16));
#37164=CARTESIAN_POINT('',(29.470836477965,-3.9278981228736,0.00143380487199485));
#37165=CARTESIAN_POINT('',(23.75,-3.933,-4.81653586104654E-16));
#37166=CARTESIAN_POINT('',(29.567,-3.56151197810526,1.66856867698419));
#37167=CARTESIAN_POINT('Origin',(29.567,0.,0.));
#37168=CARTESIAN_POINT('Ctrl Pts',(29.567,-3.56151197810523,1.66856867698424));
#37169=CARTESIAN_POINT('Ctrl Pts',(29.5015515681492,-3.01258675481066,2.84023382017821));
#37170=CARTESIAN_POINT('Ctrl Pts',(29.4361031362984,-1.84538537124581,3.71044748004995));
#37171=CARTESIAN_POINT('Ctrl Pts',(29.3706547044477,-0.572813470363568,
3.89689459583817));
#37172=CARTESIAN_POINT('Ctrl Pts',(29.3052062725969,0.699758430518651,4.08334171162639));
#37173=CARTESIAN_POINT('Ctrl Pts',(29.2397578407461,2.07770084871824,3.58602228333111));
#37174=CARTESIAN_POINT('Ctrl Pts',(29.1743094088954,2.93709163106757,2.62598383516187));
#37175=CARTESIAN_POINT('Ctrl Pts',(29.1088609770446,3.79648241341692,1.66594538699262));
#37176=CARTESIAN_POINT('Ctrl Pts',(29.0434125451938,4.13732155991598,0.243187918949396));
#37177=CARTESIAN_POINT('Ctrl Pts',(28.977964113343,3.80910353312742,-1.00277003521058));
#37178=CARTESIAN_POINT('Ctrl Pts',(28.9125156814922,3.48088550633886,-2.24872798937053));
#37179=CARTESIAN_POINT('Ctrl Pts',(28.8470672496415,2.48361030626269,-3.31788642964727));
#37180=CARTESIAN_POINT('Ctrl Pts',(28.7816188177907,1.26359152250731,-3.73099214383412));
#37181=CARTESIAN_POINT('Ctrl Pts',(28.7161703859399,0.0435727387519015,
-4.14409785802099));
#37182=CARTESIAN_POINT('Ctrl Pts',(28.6507219540891,-1.39918962868272,-3.90115084611797));
#37183=CARTESIAN_POINT('Ctrl Pts',(28.5852735222384,-2.41662917135091,-3.11089977775168));
#37184=CARTESIAN_POINT('Ctrl Pts',(28.5249035221706,-3.35512110344034,-2.38196776667424));
#37185=CARTESIAN_POINT('Ctrl Pts',(28.4645335221028,-3.93173472701253,-1.1873719006031));
#37186=CARTESIAN_POINT('Ctrl Pts',(28.404163522035,-3.93818417569795,0.00170700930730246));
#37187=CARTESIAN_POINT('Ctrl Pts',(28.220836477965,-3.93866152695812,0.00124115044389661));
#37188=CARTESIAN_POINT('Ctrl Pts',(28.2826578734011,-3.93356747382553,-1.21603278132397));
#37189=CARTESIAN_POINT('Ctrl Pts',(28.3444792688372,-3.32498523962417,-2.4377239649422));
#37190=CARTESIAN_POINT('Ctrl Pts',(28.4063006642733,-2.34789226689304,-3.16300368438513));
#37191=CARTESIAN_POINT('Ctrl Pts',(28.4717490961241,-1.31347364229616,-3.93083527336599));
#37192=CARTESIAN_POINT('Ctrl Pts',(28.5371975279749,0.133964933385241,-4.14229816744944));
#37193=CARTESIAN_POINT('Ctrl Pts',(28.6026459598256,1.34479136791605,-3.70252107236144));
#37194=CARTESIAN_POINT('Ctrl Pts',(28.6680943916764,2.55561780244685,-3.26274397727345));
#37195=CARTESIAN_POINT('Ctrl Pts',(28.7335428235272,3.52983209582705,-2.17172689301403));
#37196=CARTESIAN_POINT('Ctrl Pts',(28.798991255378,3.83042460753331,-0.919022093761055));
#37197=CARTESIAN_POINT('Ctrl Pts',(28.8644396872287,4.13101711923956,0.333682705491934));
#37198=CARTESIAN_POINT('Ctrl Pts',(28.9298881190795,3.75798784927184,1.7480752197385));
#37199=CARTESIAN_POINT('Ctrl Pts',(28.9953365509303,2.87839874358939,2.68935253297113));
#37200=CARTESIAN_POINT('Ctrl Pts',(29.0607849827811,1.99880963790694,3.63062984620376));
#37201=CARTESIAN_POINT('Ctrl Pts',(29.1262334146319,0.612660696509772,4.09879195842248));
#37202=CARTESIAN_POINT('Ctrl Pts',(29.1916818464826,-0.657352822470509,
3.88392269629536));
#37203=CARTESIAN_POINT('Ctrl Pts',(29.2571302783334,-1.92736634145081,3.66905343416824));
#37204=CARTESIAN_POINT('Ctrl Pts',(29.3225787101841,-3.0812444380142,2.77115279769526));
#37205=CARTESIAN_POINT('Ctrl Pts',(29.3880271420349,-3.60246465164686,1.59281990421752));
#37206=CARTESIAN_POINT('Ctrl Pts',(29.4156302540116,-3.8222911549651,1.095853760267));
#37207=CARTESIAN_POINT('Ctrl Pts',(29.4432333659883,-3.92958294012511,0.54900541954638));
#37208=CARTESIAN_POINT('Ctrl Pts',(29.470836477965,-3.9278981228736,0.00143380487199485));
#37209=CARTESIAN_POINT('Origin',(15.6892265507269,0.,0.));
#37210=CARTESIAN_POINT('',(28.8142265507269,-3.2269979792094,0.00139874504058523));
#37211=CARTESIAN_POINT('',(29.0607734492731,-3.2185694572822,0.00117487786690768));
#37212=CARTESIAN_POINT('',(15.6892265507269,-3.22275,-1.83004677902795E-13));
#37213=CARTESIAN_POINT('',(29.567,2.58354504679088,1.93441189848628));
#37214=CARTESIAN_POINT('Ctrl Pts',(28.8142265507269,-3.2269979792094,0.00139874504058531));
#37215=CARTESIAN_POINT('Ctrl Pts',(28.8745965507947,-3.22171321929302,-0.972947569964154));
#37216=CARTESIAN_POINT('Ctrl Pts',(29.0004149827133,-2.23699797382901,-3.01302555875835));
#37217=CARTESIAN_POINT('Ctrl Pts',(29.1916818464826,1.21792180611816,-3.59480011557272));
#37218=CARTESIAN_POINT('Ctrl Pts',(29.3822363295059,3.5971583139091,-1.04406909014969));
#37219=CARTESIAN_POINT('Ctrl Pts',(29.5073423806783,3.15601612891197,1.15992870617642));
#37220=CARTESIAN_POINT('Ctrl Pts',(29.567,2.58354504679088,1.93441189848628));
#37221=CARTESIAN_POINT('',(29.567,2.66526038810872,-1.81176836987473));
#37222=CARTESIAN_POINT('Origin',(29.567,0.,0.));
#37223=CARTESIAN_POINT('Ctrl Pts',(29.0607734492731,-3.2185694572822,0.00117487786690823));
#37224=CARTESIAN_POINT('Ctrl Pts',(29.0986187691472,-3.21667663602536,-0.613998780257283));
#37225=CARTESIAN_POINT('Ctrl Pts',(29.201912520872,-2.75336214083532,-2.29607392539308));
#37226=CARTESIAN_POINT('Ctrl Pts',(29.3706547044477,-0.0451685032330799,
-3.79409447712557));
#37227=CARTESIAN_POINT('Ctrl Pts',(29.5015515681492,2.06922537276306,-2.68858493359273));
#37228=CARTESIAN_POINT('Ctrl Pts',(29.567,2.6652603881087,-1.81176836987477));
#37229=CARTESIAN_POINT('Origin',(15.6892265507269,0.,0.));
#37230=CARTESIAN_POINT('',(27.5642265507269,-3.22109517432664,-0.0026659098327413));
#37231=CARTESIAN_POINT('',(27.8107734492731,-3.22738912687624,0.00101701438904953));
#37232=CARTESIAN_POINT('',(15.6892265507269,-3.22275,-1.83004677902795E-13));
#37233=CARTESIAN_POINT('Ctrl Pts',(27.5642265507269,-3.22109517432664,-0.00266590983274053));
#37234=CARTESIAN_POINT('Ctrl Pts',(27.5831241945059,-3.22357985231351,-0.309115529678735));
#37235=CARTESIAN_POINT('Ctrl Pts',(27.6674702701357,-3.04388313860946,-1.67404196095562));
#37236=CARTESIAN_POINT('Ctrl Pts',(27.8172647776164,-1.11763786140405,-3.62729345221592));
#37237=CARTESIAN_POINT('Ctrl Pts',(28.0136100731686,2.41032302518161,-2.93201452186437));
#37238=CARTESIAN_POINT('Ctrl Pts',(28.2099553687211,3.77496404659118,0.394752895225204));
#37239=CARTESIAN_POINT('Ctrl Pts',(28.4063006642733,1.75161877719691,3.36725853372798));
#37240=CARTESIAN_POINT('Ctrl Pts',(28.6026459598257,-1.84395765825054,3.31756249130118));
#37241=CARTESIAN_POINT('Ctrl Pts',(28.7386212553102,-3.18770250249994,1.22119202818211));
#37242=CARTESIAN_POINT('Ctrl Pts',(28.8091481189439,-3.22744254261332,0.0833624900826931));
#37243=CARTESIAN_POINT('Ctrl Pts',(28.8142265507269,-3.2269979792094,0.00139874504058531));
#37244=CARTESIAN_POINT('Ctrl Pts',(27.8107734492731,-3.22738912687624,0.00101701438904955));
#37245=CARTESIAN_POINT('Ctrl Pts',(27.8725948447092,-3.22321499523797,-0.996432658533559));
#37246=CARTESIAN_POINT('Ctrl Pts',(27.9998646719961,-2.19659766354631,-3.05730343752226));
#37247=CARTESIAN_POINT('Ctrl Pts',(28.1925829311337,1.2958220592028,-3.56752694153447));
#37248=CARTESIAN_POINT('Ctrl Pts',(28.388928226686,3.69067264195723,-0.885547301338346));
#37249=CARTESIAN_POINT('Ctrl Pts',(28.5852735222384,2.77367792053198,2.59136610467845));
#37250=CARTESIAN_POINT('Ctrl Pts',(28.7816188177907,-0.633806061838565,
3.7422199926669));
#37251=CARTESIAN_POINT('Ctrl Pts',(28.9401187934689,-2.92357971927845,1.96041199187571));
#37252=CARTESIAN_POINT('Ctrl Pts',(29.0331703372964,-3.21995001787142,0.449861992332215));
#37253=CARTESIAN_POINT('Ctrl Pts',(29.0607734492731,-3.2185694572822,0.00117487786690823));
#37254=CARTESIAN_POINT('Origin',(15.6892265507269,0.,0.));
#37255=CARTESIAN_POINT('',(26.3142265507269,-3.21963434354893,0.00223887197271718));
#37256=CARTESIAN_POINT('',(26.5607734492731,-3.22048443636447,-0.00253212360901173));
#37257=CARTESIAN_POINT('',(15.6892265507269,-3.22275,-1.83004677902795E-13));
#37258=CARTESIAN_POINT('Ctrl Pts',(26.3142265507269,-3.21963434354893,0.00223887197271691));
#37259=CARTESIAN_POINT('Ctrl Pts',(26.3571002700679,-3.21505606815715,-0.693813677238957));
#37260=CARTESIAN_POINT('Ctrl Pts',(26.4654224212598,-2.65391429960236,-2.45914715185642));
#37261=CARTESIAN_POINT('Ctrl Pts',(26.6391930043024,0.237686884393074,-3.7881193692251));
#37262=CARTESIAN_POINT('Ctrl Pts',(26.8355382998547,3.29161350856939,-1.88987422206122));
#37263=CARTESIAN_POINT('Ctrl Pts',(27.0318835954071,3.39129182252066,1.70454680934583));
#37264=CARTESIAN_POINT('Ctrl Pts',(27.2282288909593,0.447261799442319,3.76912497394121));
#37265=CARTESIAN_POINT('Ctrl Pts',(27.4056765427327,-2.57620177321888,2.57776097278147));
#37266=CARTESIAN_POINT('Ctrl Pts',(27.5176757626552,-3.21497463783302,0.752215041195907));
#37267=CARTESIAN_POINT('Ctrl Pts',(27.5642265507269,-3.22109517432664,-0.00266590983274053));
#37268=CARTESIAN_POINT('Ctrl Pts',(26.5607734492731,-3.22048443636446,-0.002532123609012));
#37269=CARTESIAN_POINT('Ctrl Pts',(26.5811224884204,-3.22298870685491,-0.332677235491898));
#37270=CARTESIAN_POINT('Ctrl Pts',(26.6669199594186,-3.02559276303903,-1.72174377610718));
#37271=CARTESIAN_POINT('Ctrl Pts',(26.8181658622674,-1.03798327082204,-3.65088212414849));
#37272=CARTESIAN_POINT('Ctrl Pts',(27.0145111578197,2.47390373029963,-2.87856768367053));
#37273=CARTESIAN_POINT('Ctrl Pts',(27.2108564533721,3.76543843873028,0.477281287863921));
#37274=CARTESIAN_POINT('Ctrl Pts',(27.4072017489244,1.67747438921608,3.40476947033153));
#37275=CARTESIAN_POINT('Ctrl Pts',(27.6035470444767,-1.91605542660869,3.27644640572374));
#37276=CARTESIAN_POINT('Ctrl Pts',(27.738070944593,-3.19988118387297,1.17378932561218));
#37277=CARTESIAN_POINT('Ctrl Pts',(27.8071464128584,-3.22763402150124,0.0595369856705937));
#37278=CARTESIAN_POINT('Ctrl Pts',(27.8107734492731,-3.22738912687624,0.00101701438904955));
#37279=CARTESIAN_POINT('Origin',(15.6892265507269,0.,0.));
#37280=CARTESIAN_POINT('',(25.0642265507269,-3.22774412020477,-0.000401821292809558));
#37281=CARTESIAN_POINT('',(25.3107734492731,-3.22017561685325,0.00244165668128279));
#37282=CARTESIAN_POINT('',(15.6892265507269,-3.22275,-1.83004677902795E-13));
#37283=CARTESIAN_POINT('Ctrl Pts',(25.0642265507269,-3.22774412020477,-0.000401821292809641));
#37284=CARTESIAN_POINT('Ctrl Pts',(25.0656279137792,-3.22778459631103,-0.0230053114811701));
#37285=CARTESIAN_POINT('Ctrl Pts',(25.1324777086823,-3.21741583386448,-1.10123077018649));
#37286=CARTESIAN_POINT('Ctrl Pts',(25.2647759354361,-2.02490994382068,-3.2103088390008));
#37287=CARTESIAN_POINT('Ctrl Pts',(25.4611212309884,1.56227329051694,-3.45913938637011));
#37288=CARTESIAN_POINT('Ctrl Pts',(25.6574665265407,3.74730462149625,-0.603366577456954));
#37289=CARTESIAN_POINT('Ctrl Pts',(25.8538118220931,2.56910214256522,2.79393222142319));
#37290=CARTESIAN_POINT('Ctrl Pts',(26.0501571176454,-0.914888612658763,
3.68365606078035));
#37291=CARTESIAN_POINT('Ctrl Pts',(26.2036286938567,-2.99629870821356,1.79491000424181));
#37292=CARTESIAN_POINT('Ctrl Pts',(26.2916518382172,-3.22204498700017,0.368738126798843));
#37293=CARTESIAN_POINT('Ctrl Pts',(26.3142265507269,-3.21963434354893,0.00223887197271691));
#37294=CARTESIAN_POINT('Ctrl Pts',(25.3107734492731,-3.22017561685325,0.00244165668128262));
#37295=CARTESIAN_POINT('Ctrl Pts',(25.3550985639825,-3.21495240151903,-0.716868791691903));
#37296=CARTESIAN_POINT('Ctrl Pts',(25.4648721105426,-2.62384997733627,-2.50606997404072));
#37297=CARTESIAN_POINT('Ctrl Pts',(25.6400940889534,0.320532234955617,-3.78201078961425));
#37298=CARTESIAN_POINT('Ctrl Pts',(25.8364393845058,3.33218487481924,-1.81738565586481));
#37299=CARTESIAN_POINT('Ctrl Pts',(26.0327846800581,3.353176683897,1.77835660933565));
#37300=CARTESIAN_POINT('Ctrl Pts',(26.2291299756105,0.364667642181413,3.7780106271763));
#37301=CARTESIAN_POINT('Ctrl Pts',(26.4051262320154,-2.60748720280079,2.53104817443241));
#37302=CARTESIAN_POINT('Ctrl Pts',(26.5156740565697,-3.21493424416785,0.729165522757876));
#37303=CARTESIAN_POINT('Ctrl Pts',(26.5607734492731,-3.22048443636446,-0.002532123609012));
#37304=CARTESIAN_POINT('Origin',(15.6892265507269,0.,0.));
#37305=CARTESIAN_POINT('',(23.8142265507269,-3.21875508197893,-0.00173903194394261));
#37306=CARTESIAN_POINT('',(24.0607734492731,-3.22754701096656,-0.000807333834090818));
#37307=CARTESIAN_POINT('',(15.6892265507269,-3.22275,-1.83004677902795E-13));
#37308=CARTESIAN_POINT('Ctrl Pts',(23.8142265507269,-3.21875508197893,-0.00173903194394299));
#37309=CARTESIAN_POINT('Ctrl Pts',(23.8396039893412,-3.22082245996468,-0.414024034281807));
#37310=CARTESIAN_POINT('Ctrl Pts',(23.9304298598063,-2.95721982843924,-1.88704958033111));
#37311=CARTESIAN_POINT('Ctrl Pts',(24.0867041621221,-0.758431521083658,
-3.71902201613955));
#37312=CARTESIAN_POINT('Ctrl Pts',(24.2830494576745,2.68485587331004,-2.68288875433691));
#37313=CARTESIAN_POINT('Ctrl Pts',(24.4793947532267,3.71846513208049,0.761157139313524));
#37314=CARTESIAN_POINT('Ctrl Pts',(24.6757400487791,1.41472424965457,3.52205883332719));
#37315=CARTESIAN_POINT('Ctrl Pts',(24.8706839812791,-2.13323749993867,3.12474262705387));
#37316=CARTESIAN_POINT('Ctrl Pts',(25.0001794819284,-3.22589422416346,1.03265473662003));
#37317=CARTESIAN_POINT('Ctrl Pts',(25.0642265507269,-3.22774412020477,-0.000401821292809641));
#37318=CARTESIAN_POINT('Ctrl Pts',(24.0607734492731,-3.22754701096656,-0.000807333834090818));
#37319=CARTESIAN_POINT('Ctrl Pts',(24.0636262076937,-3.22770425869004,-0.0468288853761836));
#37320=CARTESIAN_POINT('Ctrl Pts',(24.131927397965,-3.20613122516383,-1.14853352224944));
#37321=CARTESIAN_POINT('Ctrl Pts',(24.2656770200872,-1.95416830672108,-3.25385505757741));
#37322=CARTESIAN_POINT('Ctrl Pts',(24.4620223156395,1.63760182067,-3.42412131560862));
#37323=CARTESIAN_POINT('Ctrl Pts',(24.6583676111919,3.75961212255236,-0.521213199180538));
#37324=CARTESIAN_POINT('Ctrl Pts',(24.8547129067441,2.50734255139624,2.84948764361036));
#37325=CARTESIAN_POINT('Ctrl Pts',(25.0510582022965,-0.995285623997665,
3.66275211200675));
#37326=CARTESIAN_POINT('Ctrl Pts',(25.2030783831395,-3.01557416881359,1.74719555501021));
#37327=CARTESIAN_POINT('Ctrl Pts',(25.2896501321317,-3.22266476177089,0.345232032380632));
#37328=CARTESIAN_POINT('Ctrl Pts',(25.3107734492731,-3.22017561685325,0.00244165668128262));
#37329=CARTESIAN_POINT('Origin',(15.6892265507269,0.,0.));
#37330=CARTESIAN_POINT('',(22.5642265507269,-3.22236731757899,0.00278473722726826));
#37331=CARTESIAN_POINT('',(22.8107734492731,-3.21839779706106,-0.00143350544814236));
#37332=CARTESIAN_POINT('',(15.6892265507269,-3.22275,-1.83004677902795E-13));
#37333=CARTESIAN_POINT('Ctrl Pts',(22.5642265507269,-3.22236731757899,0.00278473722726828));
#37334=CARTESIAN_POINT('Ctrl Pts',(22.6135800649032,-3.2153580953679,-0.796740891757197));
#37335=CARTESIAN_POINT('Ctrl Pts',(22.7283820109303,-2.5134926350336,-2.66752532507124));
#37336=CARTESIAN_POINT('Ctrl Pts',(22.9086323888082,0.606112968189978,-3.74686138016046));
#37337=CARTESIAN_POINT('Ctrl Pts',(23.1049776843605,3.46028350989628,-1.55973752903206));
#37338=CARTESIAN_POINT('Ctrl Pts',(23.3013229799128,3.2088238385529,2.02726236612665));
#37339=CARTESIAN_POINT('Ctrl Pts',(23.4976682754651,0.0774208817006576,
3.79477919467037));
#37340=CARTESIAN_POINT('Ctrl Pts',(23.6686361324032,-2.709756129895,2.36820545374654));
#37341=CARTESIAN_POINT('Ctrl Pts',(23.7741555574904,-3.21549069070038,0.649259273727197));
#37342=CARTESIAN_POINT('Ctrl Pts',(23.8142265507269,-3.21875508197893,-0.00173903194394299));
#37343=CARTESIAN_POINT('Ctrl Pts',(22.8107734492731,-3.21839779706106,-0.00143350544814225));
#37344=CARTESIAN_POINT('Ctrl Pts',(22.8376022832557,-3.22018694967564,-0.437419828459572));
#37345=CARTESIAN_POINT('Ctrl Pts',(22.9298795490891,-2.93600293487459,-1.93475253165454));
#37346=CARTESIAN_POINT('Ctrl Pts',(23.0876052467732,-0.676859980052826,
-3.73472985306225));
#37347=CARTESIAN_POINT('Ctrl Pts',(23.2839505423255,2.7429275988463,-2.62348903081641));
#37348=CARTESIAN_POINT('Ctrl Pts',(23.4802958378779,3.70091723594858,0.842352729023196));
#37349=CARTESIAN_POINT('Ctrl Pts',(23.6766411334301,1.33730609950109,3.55217664308397));
#37350=CARTESIAN_POINT('Ctrl Pts',(23.870133670562,-2.17476694705372,3.080844659123));
#37351=CARTESIAN_POINT('Ctrl Pts',(23.9981777758429,-3.2240966567144,1.00900478004714));
#37352=CARTESIAN_POINT('Ctrl Pts',(24.0607734492731,-3.22754701096656,-0.000807333834090818));
#37353=CARTESIAN_POINT('Origin',(15.6892265507269,0.,0.));
#37354=CARTESIAN_POINT('',(21.3142265507269,-3.22607546549254,-0.00200277449169663));
#37355=CARTESIAN_POINT('',(21.5607734492731,-3.22305249003289,0.00276936624546656));
#37356=CARTESIAN_POINT('',(15.6892265507269,-3.22275,-1.83004677902795E-13));
#37357=CARTESIAN_POINT('Ctrl Pts',(21.3142265507269,-3.22607546549254,-0.00200277449169652));
#37358=CARTESIAN_POINT('Ctrl Pts',(21.3221077086144,-3.2270099175131,-0.129297585349694));
#37359=CARTESIAN_POINT('Ctrl Pts',(21.3954372983528,-3.16284144025928,-1.31275209178423));
#37360=CARTESIAN_POINT('Ctrl Pts',(21.5342153199419,-1.70206088753426,-3.39254056088757));
#37361=CARTESIAN_POINT('Ctrl Pts',(21.7305606154942,1.89228634899218,-3.29022729579853));
#37362=CARTESIAN_POINT('Ctrl Pts',(21.9269059110465,3.78829252219229,-0.234910438249147));
#37363=CARTESIAN_POINT('Ctrl Pts',(22.1232512065989,2.28427793986952,3.03124023631671));
#37364=CARTESIAN_POINT('Ctrl Pts',(22.3195965021511,-1.26989309433504,3.57683025625195));
#37365=CARTESIAN_POINT('Ctrl Pts',(22.4665882835272,-3.07743188805749,1.58197501572629));
#37366=CARTESIAN_POINT('Ctrl Pts',(22.5481316330524,-3.22465312956892,0.26352197938507));
#37367=CARTESIAN_POINT('Ctrl Pts',(22.5642265507269,-3.22236731757899,0.00278473722726828));
#37368=CARTESIAN_POINT('Ctrl Pts',(21.5607734492731,-3.22305249003289,0.0027693662454667));
#37369=CARTESIAN_POINT('Ctrl Pts',(21.6115783588177,-3.21572847361237,-0.81982052848557));
#37370=CARTESIAN_POINT('Ctrl Pts',(21.7278317002131,-2.47981631979778,-2.713754880308));
#37371=CARTESIAN_POINT('Ctrl Pts',(21.9095334734593,0.687967117255592,-3.7326997973555));
#37372=CARTESIAN_POINT('Ctrl Pts',(22.1058787690116,3.4935896922385,-1.48363660295612));
#37373=CARTESIAN_POINT('Ctrl Pts',(22.3022240645639,3.16368950509114,2.09700148223756));
#37374=CARTESIAN_POINT('Ctrl Pts',(22.4985693601162,-0.0056455659831341,
3.79556512770198));
#37375=CARTESIAN_POINT('Ctrl Pts',(22.668085821686,-2.73754467296897,2.32096163862923));
#37376=CARTESIAN_POINT('Ctrl Pts',(22.7721538514049,-3.21582234579305,0.626160540631221));
#37377=CARTESIAN_POINT('Ctrl Pts',(22.8107734492731,-3.21839779706106,-0.00143350544814225));
#37378=CARTESIAN_POINT('Origin',(15.6892265507269,0.,0.));
#37379=CARTESIAN_POINT('',(20.0642265507269,-3.21774602634612,-0.000218779794079732));
#37380=CARTESIAN_POINT('',(20.3107734492731,-3.22548804594158,-0.00225964513658777));
#37381=CARTESIAN_POINT('',(15.6892265507269,-3.22275,-1.83004677902795E-13));
#37382=CARTESIAN_POINT('Ctrl Pts',(20.0642265507269,-3.21774602634612,-0.000218779794079575));
#37383=CARTESIAN_POINT('Ctrl Pts',(20.0960837841765,-3.21806969513006,-0.518183692896789));
#37384=CARTESIAN_POINT('Ctrl Pts',(20.1933894494768,-2.85716533250164,-2.09984699965927));
#37385=CARTESIAN_POINT('Ctrl Pts',(20.3561435466279,-0.391994200717362,
-3.77526967626554));
#37386=CARTESIAN_POINT('Ctrl Pts',(20.5524888421802,2.93378458769563,-2.4081644931002));
#37387=CARTESIAN_POINT('Ctrl Pts',(20.7488341377326,3.62647114324965,1.12029158418925));
#37388=CARTESIAN_POINT('Ctrl Pts',(20.9451794332849,1.06437219164148,3.64327488510088));
#37389=CARTESIAN_POINT('Ctrl Pts',(21.1336435709497,-2.31182328174945,2.92637254547445));
#37390=CARTESIAN_POINT('Ctrl Pts',(21.2566592767637,-3.21924983704549,0.927811772471571));
#37391=CARTESIAN_POINT('Ctrl Pts',(21.3142265507269,-3.22607546549254,-0.00200277449169652));
#37392=CARTESIAN_POINT('Ctrl Pts',(20.3107734492731,-3.22548804594158,-0.00225964513658772));
#37393=CARTESIAN_POINT('Ctrl Pts',(20.320106002529,-3.22669615753964,-0.153069114623829));
#37394=CARTESIAN_POINT('Ctrl Pts',(20.3948869876356,-3.14910495911347,-1.36024458870627));
#37395=CARTESIAN_POINT('Ctrl Pts',(20.5351164045929,-1.62740828908083,-3.42897735581699));
#37396=CARTESIAN_POINT('Ctrl Pts',(20.7314617001453,1.96383919998109,-3.24802756047599));
#37397=CARTESIAN_POINT('Ctrl Pts',(20.9278069956976,3.79252667009079,-0.151948165376663));
#37398=CARTESIAN_POINT('Ctrl Pts',(21.12415229125,2.21739307147785,3.08050548935726));
#37399=CARTESIAN_POINT('Ctrl Pts',(21.3204975868023,-1.34786724289322,3.5481827119883));
#37400=CARTESIAN_POINT('Ctrl Pts',(21.46603797281,-3.09390410280276,1.53433044604769));
#37401=CARTESIAN_POINT('Ctrl Pts',(21.5461299269669,-3.22516349463433,0.239864827693846));
#37402=CARTESIAN_POINT('Ctrl Pts',(21.5607734492731,-3.22305249003289,0.0027693662454667));
#37403=CARTESIAN_POINT('Origin',(15.6892265507269,0.,0.));
#37404=CARTESIAN_POINT('',(18.8142265507269,-3.22532168306538,0.00249477058570468));
#37405=CARTESIAN_POINT('',(19.0607734492731,-3.21773234909139,0.000164702477305489));
#37406=CARTESIAN_POINT('',(15.6892265507269,-3.22275,-1.83004677902795E-13));
#37407=CARTESIAN_POINT('Ctrl Pts',(18.8142265507269,-3.22532168306538,0.00249477058570481));
#37408=CARTESIAN_POINT('Ctrl Pts',(18.8700598597385,-3.21799059361425,-0.899808200435379));
#37409=CARTESIAN_POINT('Ctrl Pts',(18.9913416006008,-2.35673079795164,-2.87262221235205));
#37410=CARTESIAN_POINT('Ctrl Pts',(19.178071773314,0.968794511424788,-3.66969878371352));
#37411=CARTESIAN_POINT('Ctrl Pts',(19.3744170688663,3.59592225045646,-1.21480199941451));
#37412=CARTESIAN_POINT('Ctrl Pts',(19.5707623644186,2.99575257360889,2.33067906227099));
#37413=CARTESIAN_POINT('Ctrl Pts',(19.7671076599709,-0.293163078231386,
3.78420913942485));
#37414=CARTESIAN_POINT('Ctrl Pts',(19.9315957220737,-2.8280080972332,2.15667308312832));
#37415=CARTESIAN_POINT('Ctrl Pts',(20.0306353523257,-3.2174047405168,0.545938569005431));
#37416=CARTESIAN_POINT('Ctrl Pts',(20.0642265507269,-3.21774602634612,-0.000218779794079575));
#37417=CARTESIAN_POINT('Ctrl Pts',(19.0607734492731,-3.21773234909139,0.000164702477305698));
#37418=CARTESIAN_POINT('Ctrl Pts',(19.094082078091,-3.21750794441159,-0.541409146678799));
#37419=CARTESIAN_POINT('Ctrl Pts',(19.1928391387596,-2.8328436003506,-2.14744201793394));
#37420=CARTESIAN_POINT('Ctrl Pts',(19.357044631279,-0.309271563708209,-3.78292723677877));
#37421=CARTESIAN_POINT('Ctrl Pts',(19.5533899268313,2.98578041436392,-2.34339172240098));
#37422=CARTESIAN_POINT('Ctrl Pts',(19.7497352223837,3.60108775863409,1.19939252423599));
#37423=CARTESIAN_POINT('Ctrl Pts',(19.946080517936,0.984384060858174,3.66569394308102));
#37424=CARTESIAN_POINT('Ctrl Pts',(20.1330932602325,-2.34943880221939,2.88116800122945));
#37425=CARTESIAN_POINT('Ctrl Pts',(20.2546575706782,-3.21822376982043,0.904545346885408));
#37426=CARTESIAN_POINT('Ctrl Pts',(20.3107734492731,-3.22548804594158,-0.00225964513658772));
#37427=CARTESIAN_POINT('Origin',(1.07322330470336,0.,-2.95337249083895E-16));
#37428=CARTESIAN_POINT('',(1.5,10.,-1.22464679914735E-15));
#37429=CARTESIAN_POINT('',(1.5,-10.,-1.22464679914735E-15));
#37430=CARTESIAN_POINT('Origin',(1.5,0.,0.));
#37431=CARTESIAN_POINT('Origin',(1.5,0.,0.));
#37432=CARTESIAN_POINT('',(0.646446609406726,9.64644660940673,1.18134899633558E-15));
#37433=CARTESIAN_POINT('',(1.07322330470336,9.82322330470336,1.20299789774147E-15));
#37434=CARTESIAN_POINT('',(0.646446609406727,-9.64644660940673,-1.18134899633558E-15));
#37435=CARTESIAN_POINT('Origin',(0.646446609406726,0.,-5.90674498167789E-16));
#37436=CARTESIAN_POINT('Origin',(0.646446609406726,0.,-5.90674498167789E-16));
#37437=CARTESIAN_POINT('Origin',(0.499999999999998,0.,0.));
#37438=CARTESIAN_POINT('',(0.353553390593272,-9.35355339059327,-1.14547992204439E-15));
#37439=CARTESIAN_POINT('',(0.499999999999998,-9.5,-1.16341445918999E-15));
#37440=CARTESIAN_POINT('',(0.353553390593273,9.35355339059327,-1.14547992204439E-15));
#37441=CARTESIAN_POINT('Origin',(0.353553390593273,0.,-5.72739961022196E-16));
#37442=CARTESIAN_POINT('Origin',(0.353553390593273,0.,-5.72739961022196E-16));
#37443=CARTESIAN_POINT('Origin',(8.5,0.,0.));
#37444=CARTESIAN_POINT('',(16.,-10.,-1.22464679914735E-15));
#37445=CARTESIAN_POINT('Origin',(16.,0.,0.));
#37446=CARTESIAN_POINT('',(8.5,-10.,-1.22464679914735E-15));
#37447=CARTESIAN_POINT('Origin',(0.176776695296637,0.,-2.86369980511098E-16));
#37448=CARTESIAN_POINT('',(0.,8.5,1.04094977927525E-15));
#37449=CARTESIAN_POINT('',(0.176776695296637,8.92677669529664,1.09321485065982E-15));
#37450=CARTESIAN_POINT('Origin',(0.,0.,0.));
#37451=CARTESIAN_POINT('Origin',(0.,9.,0.));
#37452=CARTESIAN_POINT('Origin',(29.567,5.160062080289E-16,2.1385152528819E-16));
#37453=CARTESIAN_POINT('Ctrl Pts',(29.567,2.58354504679086,1.93441189848631));
#37454=CARTESIAN_POINT('Ctrl Pts',(29.567,2.5357479655558,2.01606960699232));
#37455=CARTESIAN_POINT('Ctrl Pts',(29.567,2.48426441181918,2.09531344700358));
#37456=CARTESIAN_POINT('Ctrl Pts',(29.567,2.42916068607862,2.17185484687615));
#37457=CARTESIAN_POINT('Ctrl Pts',(29.567,2.3689342927271,2.25551184818501));
#37458=CARTESIAN_POINT('Ctrl Pts',(29.567,2.3043843778012,2.33594190953952));
#37459=CARTESIAN_POINT('Ctrl Pts',(29.567,2.23590045951489,2.41306308144303));
#37460=CARTESIAN_POINT('Ctrl Pts',(29.567,2.19338902603406,2.4609360953035));
#37461=CARTESIAN_POINT('Ctrl Pts',(29.567,2.14936068361547,2.50753370779899));
#37462=CARTESIAN_POINT('Ctrl Pts',(29.567,2.10389981603521,2.55283175212573));
#37463=CARTESIAN_POINT('Ctrl Pts',(29.567,2.08961950353059,2.56706091807141));
#37464=CARTESIAN_POINT('Ctrl Pts',(29.567,2.07519779339987,2.58116182233106));
#37465=CARTESIAN_POINT('Ctrl Pts',(29.567,2.06063718025006,2.59513363350206));
#37466=CARTESIAN_POINT('Ctrl Pts',(29.567,2.04725437029449,2.60797526947665));
#37467=CARTESIAN_POINT('Ctrl Pts',(29.567,2.03376144273307,2.62070091822984));
#37468=CARTESIAN_POINT('Ctrl Pts',(29.567,2.02016096074622,2.63330999588553));
#37469=CARTESIAN_POINT('Ctrl Pts',(29.567,1.94243338502426,2.70537163599613));
#37470=CARTESIAN_POINT('Ctrl Pts',(29.567,1.86119439665059,2.77362993398164));
#37471=CARTESIAN_POINT('Ctrl Pts',(29.567,1.7768536571144,2.8380012403174));
#37472=CARTESIAN_POINT('Ctrl Pts',(29.567,1.6954072541691,2.90016350475531));
#37473=CARTESIAN_POINT('Ctrl Pts',(29.567,1.61106755085086,2.95870120222006));
#37474=CARTESIAN_POINT('Ctrl Pts',(29.567,1.52416618420263,3.01351548305743));
#37475=CARTESIAN_POINT('Ctrl Pts',(29.567,1.48476950634889,3.03836550150048));
#37476=CARTESIAN_POINT('Ctrl Pts',(29.567,1.4448458926919,3.0624499158597));
#37477=CARTESIAN_POINT('Ctrl Pts',(29.567,1.40442422564169,3.08575765411971));
#37478=CARTESIAN_POINT('Ctrl Pts',(29.567,1.3882956126443,3.09505765379002));
#37479=CARTESIAN_POINT('Ctrl Pts',(29.567,1.37208617296854,3.10423482964628));
#37480=CARTESIAN_POINT('Ctrl Pts',(29.567,1.35580246527857,3.11328577356711));
#37481=CARTESIAN_POINT('Ctrl Pts',(29.567,1.25886714739215,3.16716515674211));
#37482=CARTESIAN_POINT('Ctrl Pts',(29.567,1.15956514623483,3.21642936845675));
#37483=CARTESIAN_POINT('Ctrl Pts',(29.567,1.05833049025747,3.26099255600975));
#37484=CARTESIAN_POINT('Ctrl Pts',(29.567,0.955355806808139,3.30632169836185));
#37485=CARTESIAN_POINT('Ctrl Pts',(29.567,0.85038079758029,3.34678738341505));
#37486=CARTESIAN_POINT('Ctrl Pts',(29.567,0.743820340173551,3.3822652553553));
#37487=CARTESIAN_POINT('Ctrl Pts',(29.567,0.637179374181623,3.41776993154682));
#37488=CARTESIAN_POINT('Ctrl Pts',(29.567,0.528949752068905,3.44827974859085));
#37489=CARTESIAN_POINT('Ctrl Pts',(29.567,0.419516975660503,3.47362849800319));
#37490=CARTESIAN_POINT('Ctrl Pts',(29.567,0.342210256475242,3.49153564352972));
#37491=CARTESIAN_POINT('Ctrl Pts',(29.567,0.264302453480718,3.50686633363735));
#37492=CARTESIAN_POINT('Ctrl Pts',(29.567,0.185923742235531,3.51954741773577));
#37493=CARTESIAN_POINT('Ctrl Pts',(29.567,0.162525512979304,3.5233330746857));
#37494=CARTESIAN_POINT('Ctrl Pts',(29.567,0.139085294911744,3.52688251402397));
#37495=CARTESIAN_POINT('Ctrl Pts',(29.567,0.115606504489892,3.53019355998364));
#37496=CARTESIAN_POINT('Ctrl Pts',(29.567,0.0954384156821029,3.5330377213634));
#37497=CARTESIAN_POINT('Ctrl Pts',(29.567,0.0752384615584927,3.53570630508463));
#37498=CARTESIAN_POINT('Ctrl Pts',(29.567,0.0550345809701694,3.53819496903935));
#37499=CARTESIAN_POINT('Ctrl Pts',(29.567,-0.0599756574808101,3.552361645268));
#37500=CARTESIAN_POINT('Ctrl Pts',(29.567,-0.175272224620941,3.5607264093425));
#37501=CARTESIAN_POINT('Ctrl Pts',(29.567,-0.290425098911766,3.56316203636081));
#37502=CARTESIAN_POINT('Ctrl Pts',(29.567,-0.36815124373659,3.56480604133706));
#37503=CARTESIAN_POINT('Ctrl Pts',(29.567,-0.445812651568658,3.56374789754405));
#37504=CARTESIAN_POINT('Ctrl Pts',(29.567,-0.523283233678614,3.55993654290422));
#37505=CARTESIAN_POINT('Ctrl Pts',(29.567,-0.63435909064238,3.55447189463025));
#37506=CARTESIAN_POINT('Ctrl Pts',(29.567,-0.74504273400306,3.54335004573931));
#37507=CARTESIAN_POINT('Ctrl Pts',(29.567,-0.85505603383999,3.52683910178606));
#37508=CARTESIAN_POINT('Ctrl Pts',(29.567,-0.967076221847354,3.51002696135791));
#37509=CARTESIAN_POINT('Ctrl Pts',(29.567,-1.07840207048601,3.48762718741913));
#37510=CARTESIAN_POINT('Ctrl Pts',(29.567,-1.18874066520512,3.45986878136783));
#37511=CARTESIAN_POINT('Ctrl Pts',(29.567,-1.21464526759529,3.45335183710572));
#37512=CARTESIAN_POINT('Ctrl Pts',(29.567,-1.24049543083138,3.44653930625182));
#37513=CARTESIAN_POINT('Ctrl Pts',(29.567,-1.26628730485178,3.43943374373268));
#37514=CARTESIAN_POINT('Ctrl Pts',(29.567,-1.28464244035827,3.43437697419413));
#37515=CARTESIAN_POINT('Ctrl Pts',(29.567,-1.30296950645519,3.42917127609625));
#37516=CARTESIAN_POINT('Ctrl Pts',(29.567,-1.32124694883733,3.42382369155869));
#37517=CARTESIAN_POINT('Ctrl Pts',(29.567,-1.43060976561301,3.39182649546605));
#37518=CARTESIAN_POINT('Ctrl Pts',(29.567,-1.53835947619341,3.35470979815077));
#37519=CARTESIAN_POINT('Ctrl Pts',(29.567,-1.64421117916582,3.31278265355743));
#37520=CARTESIAN_POINT('Ctrl Pts',(29.567,-1.7534671731585,3.26950709228456));
#37521=CARTESIAN_POINT('Ctrl Pts',(29.567,-1.86070180847822,3.22110664138685));
#37522=CARTESIAN_POINT('Ctrl Pts',(29.567,-1.96560378724298,3.16786574642619));
#37523=CARTESIAN_POINT('Ctrl Pts',(29.567,-2.07149822315375,3.11412114975002));
#37524=CARTESIAN_POINT('Ctrl Pts',(29.567,-2.17501644885382,3.05544380388699));
#37525=CARTESIAN_POINT('Ctrl Pts',(29.567,-2.27582884554067,2.9920735879525));
#37526=CARTESIAN_POINT('Ctrl Pts',(29.567,-2.34151280990235,2.95078494546578));
#37527=CARTESIAN_POINT('Ctrl Pts',(29.567,-2.40604789877361,2.90750305324507));
#37528=CARTESIAN_POINT('Ctrl Pts',(29.567,-2.46933834269369,2.86228329757719));
#37529=CARTESIAN_POINT('Ctrl Pts',(29.567,-2.49060749325209,2.84708691512286));
#37530=CARTESIAN_POINT('Ctrl Pts',(29.567,-2.51173604271137,2.83167161394492));
#37531=CARTESIAN_POINT('Ctrl Pts',(29.567,-2.53272022923281,2.81603929283293));
#37532=CARTESIAN_POINT('Ctrl Pts',(29.567,-2.545674982638,2.80638855583869));
#37533=CARTESIAN_POINT('Ctrl Pts',(29.567,-2.55857471352845,2.79665510390201));
#37534=CARTESIAN_POINT('Ctrl Pts',(29.567,-2.57141852281522,2.78683936514258));
#37535=CARTESIAN_POINT('Ctrl Pts',(29.567,-2.58480907193538,2.77660578653097));
#37536=CARTESIAN_POINT('Ctrl Pts',(29.567,-2.59813128992878,2.76628852165279));
#37537=CARTESIAN_POINT('Ctrl Pts',(29.567,-2.61138252346487,2.75588981439117));
#37538=CARTESIAN_POINT('Ctrl Pts',(29.567,-2.70776223489835,2.68025727781063));
#37539=CARTESIAN_POINT('Ctrl Pts',(29.567,-2.80041912899082,2.60029670152484));
#37540=CARTESIAN_POINT('Ctrl Pts',(29.567,-2.88902699235769,2.51630659159321));
#37541=CARTESIAN_POINT('Ctrl Pts',(29.567,-2.9778000606268,2.43215988632824));
#37542=CARTESIAN_POINT('Ctrl Pts',(29.567,-3.0625098043098,2.34396820492412));
#37543=CARTESIAN_POINT('Ctrl Pts',(29.567,-3.14281079119611,2.25198224343805));
#37544=CARTESIAN_POINT('Ctrl Pts',(29.567,-3.2216186616731,2.16170666875852));
#37545=CARTESIAN_POINT('Ctrl Pts',(29.567,-3.29618089668985,2.06777608333632));
#37546=CARTESIAN_POINT('Ctrl Pts',(29.567,-3.36614317640108,1.97038692453017));
#37547=CARTESIAN_POINT('Ctrl Pts',(29.567,-3.43597914568637,1.87317359284375));
#37548=CARTESIAN_POINT('Ctrl Pts',(29.567,-3.50123252391352,1.7725137716817));
#37549=CARTESIAN_POINT('Ctrl Pts',(29.567,-3.56151197810524,1.66856867698424));
#37550=CARTESIAN_POINT('',(29.567,-3.48663465726742,-1.83204761571504));
#37551=CARTESIAN_POINT('Origin',(29.567,0.,0.));
#37552=CARTESIAN_POINT('Ctrl Pts',(29.567,-3.48672441430165,-1.8321351845655));
#37553=CARTESIAN_POINT('Ctrl Pts',(29.567,-3.42554918772991,-1.92852802099295));
#37554=CARTESIAN_POINT('Ctrl Pts',(29.567,-3.36004658914194,-2.02190377063076));
#37555=CARTESIAN_POINT('Ctrl Pts',(29.567,-3.29021431614292,-2.11191494002337));
#37556=CARTESIAN_POINT('Ctrl Pts',(29.567,-3.21555245835795,-2.20815126228005));
#37557=CARTESIAN_POINT('Ctrl Pts',(29.567,-3.13594084671758,-2.30054222096486));
#37558=CARTESIAN_POINT('Ctrl Pts',(29.567,-3.05179321734777,-2.3889096735599));
#37559=CARTESIAN_POINT('Ctrl Pts',(29.567,-3.00396143039123,-2.43914012209508));
#37560=CARTESIAN_POINT('Ctrl Pts',(29.567,-2.95466342451523,-2.48806976487008));
#37561=CARTESIAN_POINT('Ctrl Pts',(29.567,-2.90397163769525,-2.53565937397679));
#37562=CARTESIAN_POINT('Ctrl Pts',(29.567,-2.88322820540287,-2.55513337353872));
#37563=CARTESIAN_POINT('Ctrl Pts',(29.567,-2.86225136074878,-2.57438292681157));
#37564=CARTESIAN_POINT('Ctrl Pts',(29.567,-2.84104598347864,-2.59340510346618));
#37565=CARTESIAN_POINT('Ctrl Pts',(29.567,-2.82615821911944,-2.60676009734462));
#37566=CARTESIAN_POINT('Ctrl Pts',(29.567,-2.81116146340808,-2.619999679795));
#37567=CARTESIAN_POINT('Ctrl Pts',(29.567,-2.79606334508375,-2.63311809249039));
#37568=CARTESIAN_POINT('Ctrl Pts',(29.567,-2.70210212906268,-2.71475886272721));
#37569=CARTESIAN_POINT('Ctrl Pts',(29.567,-2.60415037276475,-2.79177128477282));
#37570=CARTESIAN_POINT('Ctrl Pts',(29.567,-2.50265605670507,-2.86397207182206));
#37571=CARTESIAN_POINT('Ctrl Pts',(29.567,-2.41384853015285,-2.92714776049014));
#37572=CARTESIAN_POINT('Ctrl Pts',(29.567,-2.32232774488169,-2.98663895631543));
#37573=CARTESIAN_POINT('Ctrl Pts',(29.567,-2.22838012565767,-3.04228906112937));
#37574=CARTESIAN_POINT('Ctrl Pts',(29.567,-2.18727804224717,-3.06663598198547));
#37575=CARTESIAN_POINT('Ctrl Pts',(29.567,-2.14571133542366,-3.09024726946961));
#37576=CARTESIAN_POINT('Ctrl Pts',(29.567,-2.10370364166454,-3.11310776922122));
#37577=CARTESIAN_POINT('Ctrl Pts',(29.567,-2.07785961441306,-3.12717203520905));
#37578=CARTESIAN_POINT('Ctrl Pts',(29.567,-2.051848672141,-3.14095210526973));
#37579=CARTESIAN_POINT('Ctrl Pts',(29.567,-2.02567630908807,-3.15444420661779));
#37580=CARTESIAN_POINT('Ctrl Pts',(29.567,-2.01068994039449,-3.16216982179608));
#37581=CARTESIAN_POINT('Ctrl Pts',(29.567,-1.99565392079183,-3.16979928816491));
#37582=CARTESIAN_POINT('Ctrl Pts',(29.567,-1.98057677496915,-3.17732840555982));
#37583=CARTESIAN_POINT('Ctrl Pts',(29.567,-1.87426334421613,-3.23041844728323));
#37584=CARTESIAN_POINT('Ctrl Pts',(29.567,-1.76579720789928,-3.2785796607992));
#37585=CARTESIAN_POINT('Ctrl Pts',(29.567,-1.65556247533349,-3.32165304965814));
#37586=CARTESIAN_POINT('Ctrl Pts',(29.567,-1.54607261710998,-3.36443538449582));
#37587=CARTESIAN_POINT('Ctrl Pts',(29.567,-1.43483710785183,-3.40219862409269));
#37588=CARTESIAN_POINT('Ctrl Pts',(29.567,-1.32222161270656,-3.43473703889271));
#37589=CARTESIAN_POINT('Ctrl Pts',(29.567,-1.21291663581304,-3.46631893331391));
#37590=CARTESIAN_POINT('Ctrl Pts',(29.567,-1.10231087406112,-3.49297866087499));
#37591=CARTESIAN_POINT('Ctrl Pts',(29.567,-0.990740369207159,-3.51447981885924));
#37592=CARTESIAN_POINT('Ctrl Pts',(29.567,-0.912857639994659,-3.52948888301319));
#37593=CARTESIAN_POINT('Ctrl Pts',(29.567,-0.834504833305636,-3.54198326314598));
#37594=CARTESIAN_POINT('Ctrl Pts',(29.567,-0.755799562093794,-3.5518679234343));
#37595=CARTESIAN_POINT('Ctrl Pts',(29.567,-0.724508003371303,-3.55579785624695));
#37596=CARTESIAN_POINT('Ctrl Pts',(29.567,-0.693160773230039,-3.55931513603026));
#37597=CARTESIAN_POINT('Ctrl Pts',(29.567,-0.661765455434889,-3.56241323914284));
#37598=CARTESIAN_POINT('Ctrl Pts',(29.567,-0.647183191863934,-3.56385222302102));
#37599=CARTESIAN_POINT('Ctrl Pts',(29.567,-0.632593320301258,-3.56520046326365));
#37600=CARTESIAN_POINT('Ctrl Pts',(29.567,-0.618005027399725,-3.56645676814378));
#37601=CARTESIAN_POINT('Ctrl Pts',(29.567,-0.506478628425292,-3.57606112420112));
#37602=CARTESIAN_POINT('Ctrl Pts',(29.567,-0.394900320726398,-3.58031092949672));
#37603=CARTESIAN_POINT('Ctrl Pts',(29.567,-0.283594313965176,-3.57902452852789));
#37604=CARTESIAN_POINT('Ctrl Pts',(29.567,-0.204277660100752,-3.57810783927324));
#37605=CARTESIAN_POINT('Ctrl Pts',(29.567,-0.125099203195263,-3.57437885322994));
#37606=CARTESIAN_POINT('Ctrl Pts',(29.567,-0.0461785851566451,-3.56775577379342));
#37607=CARTESIAN_POINT('Ctrl Pts',(29.567,0.0667712410172652,-3.55827693683443));
#37608=CARTESIAN_POINT('Ctrl Pts',(29.567,0.179194191414866,-3.54287182561656));
#37609=CARTESIAN_POINT('Ctrl Pts',(29.567,0.290735528015621,-3.52176041427356));
#37610=CARTESIAN_POINT('Ctrl Pts',(29.567,0.402570362004908,-3.5005934527257));
#37611=CARTESIAN_POINT('Ctrl Pts',(29.567,0.513519714278932,-3.47368954980131));
#37612=CARTESIAN_POINT('Ctrl Pts',(29.567,0.623196982310405,-3.44122735838397));
#37613=CARTESIAN_POINT('Ctrl Pts',(29.567,0.644440381543399,-3.43493975380889));
#37614=CARTESIAN_POINT('Ctrl Pts',(29.567,0.665635949821038,-3.42844351105179));
#37615=CARTESIAN_POINT('Ctrl Pts',(29.567,0.68678071400004,-3.42173977031026));
#37616=CARTESIAN_POINT('Ctrl Pts',(29.567,0.701774797365526,-3.41698604278281));
#37617=CARTESIAN_POINT('Ctrl Pts',(29.567,0.716742743793056,-3.41212809827565));
#37618=CARTESIAN_POINT('Ctrl Pts',(29.567,0.731670869876243,-3.40717073211752));
#37619=CARTESIAN_POINT('Ctrl Pts',(29.567,0.837287664306418,-3.37209726612978));
#37620=CARTESIAN_POINT('Ctrl Pts',(29.567,0.941079596991946,-3.33199907124987));
#37621=CARTESIAN_POINT('Ctrl Pts',(29.567,1.04272763424727,-3.28712163559775));
#37622=CARTESIAN_POINT('Ctrl Pts',(29.567,1.14450824131698,-3.24218567059793));
#37623=CARTESIAN_POINT('Ctrl Pts',(29.567,1.24414009253349,-3.1924573863102));
#37624=CARTESIAN_POINT('Ctrl Pts',(29.567,1.34127481549702,-3.13813913114634));
#37625=CARTESIAN_POINT('Ctrl Pts',(29.567,1.43724513419497,-3.08447201705832));
#37626=CARTESIAN_POINT('Ctrl Pts',(29.567,1.53077844315963,-3.02632368118162));
#37627=CARTESIAN_POINT('Ctrl Pts',(29.567,1.62150146855142,-2.96385561176368));
#37628=CARTESIAN_POINT('Ctrl Pts',(29.567,1.67545923088545,-2.92670256016997));
#37629=CARTESIAN_POINT('Ctrl Pts',(29.567,1.72842215433334,-2.88802088952323));
#37630=CARTESIAN_POINT('Ctrl Pts',(29.567,1.78030401089113,-2.84784018551755));
#37631=CARTESIAN_POINT('Ctrl Pts',(29.567,1.80469325436339,-2.82895155974546));
#37632=CARTESIAN_POINT('Ctrl Pts',(29.567,1.82884350756324,-2.80973162653502));
#37633=CARTESIAN_POINT('Ctrl Pts',(29.567,1.85274531535973,-2.79018325799309));
#37634=CARTESIAN_POINT('Ctrl Pts',(29.567,1.86456475510265,-2.78051659319429));
#37635=CARTESIAN_POINT('Ctrl Pts',(29.567,1.87631970395782,-2.77077262327817));
#37636=CARTESIAN_POINT('Ctrl Pts',(29.567,1.888003223487,-2.76095691114132));
#37637=CARTESIAN_POINT('Ctrl Pts',(29.567,1.97034400621842,-2.6917796894663));
#37638=CARTESIAN_POINT('Ctrl Pts',(29.567,2.04923212840135,-2.6189668217664));
#37639=CARTESIAN_POINT('Ctrl Pts',(29.567,2.12435271290082,-2.5427036465071));
#37640=CARTESIAN_POINT('Ctrl Pts',(29.567,2.19843508436252,-2.46749447559807));
#37641=CARTESIAN_POINT('Ctrl Pts',(29.567,2.26885383595672,-2.38892910395374));
#37642=CARTESIAN_POINT('Ctrl Pts',(29.567,2.33526556130163,-2.30715770560389));
#37643=CARTESIAN_POINT('Ctrl Pts',(29.567,2.3996396811376,-2.22789516921909));
#37644=CARTESIAN_POINT('Ctrl Pts',(29.567,2.46024915986653,-2.1456197660656));
#37645=CARTESIAN_POINT('Ctrl Pts',(29.567,2.51673667007826,-2.06045066893125));
#37646=CARTESIAN_POINT('Ctrl Pts',(29.567,2.57002707334798,-1.98010201282313));
#37647=CARTESIAN_POINT('Ctrl Pts',(29.567,2.6196488723445,-1.89717750925258));
#37648=CARTESIAN_POINT('Ctrl Pts',(29.567,2.6652603881087,-1.81176836987477));
#37649=CARTESIAN_POINT('Ctrl Pts',(17.5899369713081,-1.43290239521316,2.88667772504871));
#37650=CARTESIAN_POINT('Ctrl Pts',(17.6553854031588,-2.38256076808023,2.41528192450347));
#37651=CARTESIAN_POINT('Ctrl Pts',(17.7862822668604,-3.76505809554499,0.470670407196005));
#37652=CARTESIAN_POINT('Ctrl Pts',(17.9826275624127,-2.4662325973019,-2.88811363748521));
#37653=CARTESIAN_POINT('Ctrl Pts',(18.1789728579651,1.04930180499054,-3.6466643018069));
#37654=CARTESIAN_POINT('Ctrl Pts',(18.3753181535174,3.62142716015887,-1.1363036219263));
#37655=CARTESIAN_POINT('Ctrl Pts',(18.5716634490697,2.94414196278733,2.39593313727195));
#37656=CARTESIAN_POINT('Ctrl Pts',(18.768008744622,-0.375967469233134,3.77675880022508));
#37657=CARTESIAN_POINT('Ctrl Pts',(18.9643540401744,-3.35842001198963,1.76845082226179));
#37658=CARTESIAN_POINT('Ctrl Pts',(19.1606993357267,-3.32678023397126,-1.82732987070656));
#37659=CARTESIAN_POINT('Ctrl Pts',(19.357044631279,-0.309271563708209,-3.78292723677877));
#37660=CARTESIAN_POINT('Ctrl Pts',(19.5533899268313,2.98578041436392,-2.34339172240098));
#37661=CARTESIAN_POINT('Ctrl Pts',(19.7497352223837,3.60108775863409,1.19939252423599));
#37662=CARTESIAN_POINT('Ctrl Pts',(19.946080517936,0.984384060858174,3.66569394308102));
#37663=CARTESIAN_POINT('Ctrl Pts',(20.1424258134883,-2.5158075695727,2.84201756664935));
#37664=CARTESIAN_POINT('Ctrl Pts',(20.3387711090406,-3.75804527596442,-0.53239577264931));
#37665=CARTESIAN_POINT('Ctrl Pts',(20.5351164045929,-1.62740828908083,-3.42897735581699));
#37666=CARTESIAN_POINT('Ctrl Pts',(20.7314617001453,1.96383919998109,-3.24802756047599));
#37667=CARTESIAN_POINT('Ctrl Pts',(20.9278069956976,3.79252667009079,-0.151948165376663));
#37668=CARTESIAN_POINT('Ctrl Pts',(21.12415229125,2.21739307147785,3.08050548935726));
#37669=CARTESIAN_POINT('Ctrl Pts',(21.3204975868023,-1.34786724289322,3.5481827119883));
#37670=CARTESIAN_POINT('Ctrl Pts',(21.5168428823546,-3.70340671003476,0.831339441187419));
#37671=CARTESIAN_POINT('Ctrl Pts',(21.7131881779069,-2.73511106234691,-2.63163712022799));
#37672=CARTESIAN_POINT('Ctrl Pts',(21.9095334734593,0.687967117255592,-3.7326997973555));
#37673=CARTESIAN_POINT('Ctrl Pts',(22.1058787690116,3.4935896922385,-1.48363660295612));
#37674=CARTESIAN_POINT('Ctrl Pts',(22.3022240645639,3.16368950509114,2.09700148223756));
#37675=CARTESIAN_POINT('Ctrl Pts',(22.4985693601162,-0.0056455659831341,
3.79556512770198));
#37676=CARTESIAN_POINT('Ctrl Pts',(22.6949146556686,-3.16991370025882,2.08758081040675));
#37677=CARTESIAN_POINT('Ctrl Pts',(22.8912599512209,-3.48916068737138,-1.49402282593584));
#37678=CARTESIAN_POINT('Ctrl Pts',(23.0876052467732,-0.676859980052826,
-3.73472985306225));
#37679=CARTESIAN_POINT('Ctrl Pts',(23.2839505423255,2.7429275988463,-2.62348903081641));
#37680=CARTESIAN_POINT('Ctrl Pts',(23.4802958378779,3.70091723594858,0.842352729023196));
#37681=CARTESIAN_POINT('Ctrl Pts',(23.6766411334301,1.33730609950109,3.55217664308397));
#37682=CARTESIAN_POINT('Ctrl Pts',(23.8729864289826,-2.22654721778548,3.07389557309588));
#37683=CARTESIAN_POINT('Ctrl Pts',(24.0693317245348,-3.79205783001057,-0.163229659703893));
#37684=CARTESIAN_POINT('Ctrl Pts',(24.2656770200872,-1.95416830672108,-3.25385505757741));
#37685=CARTESIAN_POINT('Ctrl Pts',(24.4620223156395,1.63760182067,-3.42412131560862));
#37686=CARTESIAN_POINT('Ctrl Pts',(24.6583676111919,3.75961212255236,-0.521213199180538));
#37687=CARTESIAN_POINT('Ctrl Pts',(24.8547129067441,2.50734255139624,2.84948764361036));
#37688=CARTESIAN_POINT('Ctrl Pts',(25.0510582022965,-0.995285623997665,
3.66275211200675));
#37689=CARTESIAN_POINT('Ctrl Pts',(25.2474034978488,-3.6046375484147,1.18866928796936));
#37690=CARTESIAN_POINT('Ctrl Pts',(25.4437487934011,-2.97880042259369,-2.35225306850473));
#37691=CARTESIAN_POINT('Ctrl Pts',(25.6400940889534,0.320532234955617,-3.78201078961425));
#37692=CARTESIAN_POINT('Ctrl Pts',(25.8364393845058,3.33218487481924,-1.81738565586481));
#37693=CARTESIAN_POINT('Ctrl Pts',(26.0327846800581,3.353176683897,1.77835660933565));
#37694=CARTESIAN_POINT('Ctrl Pts',(26.2291299756105,0.364667642181413,3.7780106271763));
#37695=CARTESIAN_POINT('Ctrl Pts',(26.4254752711627,-2.95113369010615,2.38687188179727));
#37696=CARTESIAN_POINT('Ctrl Pts',(26.6218205667151,-3.61826984944021,-1.14650195931218));
#37697=CARTESIAN_POINT('Ctrl Pts',(26.8181658622674,-1.03798327082204,-3.65088212414849));
#37698=CARTESIAN_POINT('Ctrl Pts',(27.0145111578197,2.47390373029963,-2.87856768367053));
#37699=CARTESIAN_POINT('Ctrl Pts',(27.2108564533721,3.76543843873028,0.477281287863921));
#37700=CARTESIAN_POINT('Ctrl Pts',(27.4072017489244,1.67747438921608,3.40476947033153));
#37701=CARTESIAN_POINT('Ctrl Pts',(27.6035470444767,-1.91605542660869,3.27644640572374));
#37702=CARTESIAN_POINT('Ctrl Pts',(27.799892340029,-3.78987225417569,0.207498616647036));
#37703=CARTESIAN_POINT('Ctrl Pts',(27.9962376355814,-2.26232643032977,-3.04770082261197));
#37704=CARTESIAN_POINT('Ctrl Pts',(28.1925829311337,1.2958220592028,-3.56752694153447));
#37705=CARTESIAN_POINT('Ctrl Pts',(28.388928226686,3.69067264195723,-0.885547301338346));
#37706=CARTESIAN_POINT('Ctrl Pts',(28.5852735222384,2.77367792053198,2.59136610467845));
#37707=CARTESIAN_POINT('Ctrl Pts',(28.7816188177907,-0.633806061838565,
3.7422199926669));
#37708=CARTESIAN_POINT('Ctrl Pts',(28.977964113343,-3.47031303033562,1.53496654019299));
#37709=CARTESIAN_POINT('Ctrl Pts',(29.1743094088953,-3.19637271856563,-2.05102536576998));
#37710=CARTESIAN_POINT('Ctrl Pts',(29.3706547044477,-0.0451685032330799,
-3.79409447712557));
#37711=CARTESIAN_POINT('Ctrl Pts',(29.5015515681492,2.06922537276306,-2.68858493359273));
#37712=CARTESIAN_POINT('Ctrl Pts',(29.567,2.6652603881087,-1.81176836987477));
#37713=CARTESIAN_POINT('Ctrl Pts',(17.7266246475387,-1.53816642191913,3.09873914818277));
#37714=CARTESIAN_POINT('Ctrl Pts',(17.7920730793895,-2.55758869821535,2.59271361967877));
#37715=CARTESIAN_POINT('Ctrl Pts',(17.922969943091,-4.04164718998927,0.505246846232138));
#37716=CARTESIAN_POINT('Ctrl Pts',(18.1193152386434,-2.64740723616972,-3.10028054576993));
#37717=CARTESIAN_POINT('Ctrl Pts',(18.3156605341957,1.12638572472724,-3.91455593890342));
#37718=CARTESIAN_POINT('Ctrl Pts',(18.512005829748,3.88746482369703,-1.21977887830396));
#37719=CARTESIAN_POINT('Ctrl Pts',(18.7083511253004,3.1604248298077,2.57194342980134));
#37720=CARTESIAN_POINT('Ctrl Pts',(18.9046964208527,-0.403586831064142,
4.05420745306918));
#37721=CARTESIAN_POINT('Ctrl Pts',(19.101041716405,-3.60513661670255,1.89836494286392));
#37722=CARTESIAN_POINT('Ctrl Pts',(19.2973870119573,-3.57117251397831,-1.96156937016811));
#37723=CARTESIAN_POINT('Ctrl Pts',(19.4937323075097,-0.331991303901513,
-4.06082903595878));
#37724=CARTESIAN_POINT('Ctrl Pts',(19.690077603062,3.20512212970039,-2.51554221197617));
#37725=CARTESIAN_POINT('Ctrl Pts',(19.8864228986143,3.8656312469148,1.28750242420118));
#37726=CARTESIAN_POINT('Ctrl Pts',(20.0827681941666,1.0566989864367,3.93498353768948));
#37727=CARTESIAN_POINT('Ctrl Pts',(20.279113489719,-2.70062409027591,3.05079816052237));
#37728=CARTESIAN_POINT('Ctrl Pts',(20.4754587852713,-4.0341191939179,-0.571506686984792));
#37729=CARTESIAN_POINT('Ctrl Pts',(20.6718040808236,-1.74696112825232,-3.680877251555));
#37730=CARTESIAN_POINT('Ctrl Pts',(20.8681493763759,2.10810696217036,-3.48663450328654));
#37731=CARTESIAN_POINT('Ctrl Pts',(21.0644946719283,4.07113366385201,-0.163110597508529));
#37732=CARTESIAN_POINT('Ctrl Pts',(21.2608399674806,2.38028743488564,3.30680590813169));
#37733=CARTESIAN_POINT('Ctrl Pts',(21.4571852630329,-1.44688440828145,3.80883968415904));
#37734=CARTESIAN_POINT('Ctrl Pts',(21.6535305585853,-3.97546676390202,0.892411386793245));
#37735=CARTESIAN_POINT('Ctrl Pts',(21.8498758541376,-2.93603807933882,-2.82496272358349));
#37736=CARTESIAN_POINT('Ctrl Pts',(22.0462211496899,0.738506630097174,-4.00691178308939));
#37737=CARTESIAN_POINT('Ctrl Pts',(22.2425664452422,3.75023614624128,-1.59262767137592));
#37738=CARTESIAN_POINT('Ctrl Pts',(22.4389117407945,3.39610079679244,2.25105162603391));
#37739=CARTESIAN_POINT('Ctrl Pts',(22.6352570363469,-0.00606030114610197,
4.07439533295633));
#37740=CARTESIAN_POINT('Ctrl Pts',(22.8316023318992,-3.40278223444119,2.24093889181667));
#37741=CARTESIAN_POINT('Ctrl Pts',(23.0279476274515,-3.74548177735205,-1.60377688816228));
#37742=CARTESIAN_POINT('Ctrl Pts',(23.2242929230039,-0.726583539211172,
-4.00909097096232));
#37743=CARTESIAN_POINT('Ctrl Pts',(23.4206382185562,2.94442883506593,-2.81621605836923));
#37744=CARTESIAN_POINT('Ctrl Pts',(23.6169835141085,3.97279440780828,0.904233733940176));
#37745=CARTESIAN_POINT('Ctrl Pts',(23.8133288096608,1.43554742106091,3.81312701784159));
#37746=CARTESIAN_POINT('Ctrl Pts',(24.0096741052132,-2.39011406405363,3.29971041350562));
#37747=CARTESIAN_POINT('Ctrl Pts',(24.2060194007655,-4.07063038179243,-0.175220854160445));
#37748=CARTESIAN_POINT('Ctrl Pts',(24.4023646963179,-2.09772562473093,-3.49289010059391));
#37749=CARTESIAN_POINT('Ctrl Pts',(24.5987099918701,1.7579034981329,-3.6756644764093));
#37750=CARTESIAN_POINT('Ctrl Pts',(24.7950552874225,4.03580114435494,-0.55950261812586));
#37751=CARTESIAN_POINT('Ctrl Pts',(24.9914005829747,2.69153721404245,3.058817005064));
#37752=CARTESIAN_POINT('Ctrl Pts',(25.1877458785272,-1.06840140135594,3.93182559351093));
#37753=CARTESIAN_POINT('Ctrl Pts',(25.3840911740794,-3.86944181172621,1.27599143642233));
#37754=CARTESIAN_POINT('Ctrl Pts',(25.5804364696318,-3.19762937303946,-2.52505453122087));
#37755=CARTESIAN_POINT('Ctrl Pts',(25.7767817651841,0.344079207766316,-4.05984526465612));
#37756=CARTESIAN_POINT('Ctrl Pts',(25.9731270607364,3.5769741911216,-1.95089463236812));
#37757=CARTESIAN_POINT('Ctrl Pts',(26.1694723562888,3.59950810268922,1.9089984299113));
#37758=CARTESIAN_POINT('Ctrl Pts',(26.3658176518411,0.391456894927206,4.05555124186375));
#37759=CARTESIAN_POINT('Ctrl Pts',(26.5621629473934,-3.16793018413535,2.56221651542245));
#37760=CARTESIAN_POINT('Ctrl Pts',(26.7585082429457,-3.88407557028575,-1.23072640702519));
#37761=CARTESIAN_POINT('Ctrl Pts',(26.9548535384981,-1.11423570720934,-3.91908361135418));
#37762=CARTESIAN_POINT('Ctrl Pts',(27.1511988340504,2.65564190674782,-3.09003332609052));
#37763=CARTESIAN_POINT('Ctrl Pts',(27.3475441296027,4.04205547398569,0.512343376112075));
#37764=CARTESIAN_POINT('Ctrl Pts',(27.543889425155,1.80070518950991,3.65489100383582));
#37765=CARTESIAN_POINT('Ctrl Pts',(27.7402347207074,-2.05681289220471,3.51714105673767));
#37766=CARTESIAN_POINT('Ctrl Pts',(27.9365800162597,-4.06828424895533,0.222741901882079));
#37767=CARTESIAN_POINT('Ctrl Pts',(28.132925311812,-2.42852169287902,-3.27159134150216));
#37768=CARTESIAN_POINT('Ctrl Pts',(28.3292706073644,1.39101587582407,-3.82960498153395));
#37769=CARTESIAN_POINT('Ctrl Pts',(28.5256159029166,3.96179722437391,-0.950601470477096));
#37770=CARTESIAN_POINT('Ctrl Pts',(28.721961198469,2.9774381401227,2.78173331444731));
#37771=CARTESIAN_POINT('Ctrl Pts',(28.9183064940213,-0.680366789521514,
4.01713135199167));
#37772=CARTESIAN_POINT('Ctrl Pts',(29.1146517895737,-3.72524953174961,1.64772841386942));
#37773=CARTESIAN_POINT('Ctrl Pts',(29.310997085126,-3.43118498793819,-2.20169800725505));
#37774=CARTESIAN_POINT('Ctrl Pts',(29.5073423806783,-0.0484866765758729,
-4.07281664529234));
#37775=CARTESIAN_POINT('Ctrl Pts',(29.6382392443799,2.22123502507913,-2.88609404321281));
#37776=CARTESIAN_POINT('Ctrl Pts',(29.7036876762306,2.86105602751129,-1.94486468872292));
#37777=CARTESIAN_POINT('Ctrl Pts',(17.8633123237694,-1.6434304486251,3.31080057131684));
#37778=CARTESIAN_POINT('Ctrl Pts',(17.9287607556201,-2.73261662835048,2.77014531485408));
#37779=CARTESIAN_POINT('Ctrl Pts',(18.0596576193217,-4.31823628443353,0.539823285268273));
#37780=CARTESIAN_POINT('Ctrl Pts',(18.256002914874,-2.82858187503754,-3.31244745405465));
#37781=CARTESIAN_POINT('Ctrl Pts',(18.4523482104263,1.20346964446395,-4.18244757599994));
#37782=CARTESIAN_POINT('Ctrl Pts',(18.6486935059787,4.15350248723519,-1.30325413468162));
#37783=CARTESIAN_POINT('Ctrl Pts',(18.845038801531,3.37670769682809,2.74795372233073));
#37784=CARTESIAN_POINT('Ctrl Pts',(19.0413840970833,-0.431206192895155,
4.33165610591327));
#37785=CARTESIAN_POINT('Ctrl Pts',(19.2377293926357,-3.85185322141545,2.02827906346606));
#37786=CARTESIAN_POINT('Ctrl Pts',(19.434074688188,-3.81556479398536,-2.09580886962967));
#37787=CARTESIAN_POINT('Ctrl Pts',(19.6304199837403,-0.354711044094816,
-4.33873083513878));
#37788=CARTESIAN_POINT('Ctrl Pts',(19.8267652792926,3.42446384503687,-2.68769270155138));
#37789=CARTESIAN_POINT('Ctrl Pts',(20.023110574845,4.1301747351955,1.37561232416638));
#37790=CARTESIAN_POINT('Ctrl Pts',(20.2194558703973,1.12901391201524,4.20427313229795));
#37791=CARTESIAN_POINT('Ctrl Pts',(20.4158011659496,-2.88544061097913,3.25957875439539));
#37792=CARTESIAN_POINT('Ctrl Pts',(20.6121464615019,-4.31019311187138,-0.610617601320272));
#37793=CARTESIAN_POINT('Ctrl Pts',(20.8084917570543,-1.86651396742382,-3.932777147293));
#37794=CARTESIAN_POINT('Ctrl Pts',(21.0048370526066,2.25237472435964,-3.7252414460971));
#37795=CARTESIAN_POINT('Ctrl Pts',(21.2011823481589,4.34974065761324,-0.174273029640397));
#37796=CARTESIAN_POINT('Ctrl Pts',(21.3975276437112,2.54318179829341,3.53310632690612));
#37797=CARTESIAN_POINT('Ctrl Pts',(21.5938729392636,-1.54590157366968,4.06949665632978));
#37798=CARTESIAN_POINT('Ctrl Pts',(21.7902182348159,-4.24752681776928,0.953483332399067));
#37799=CARTESIAN_POINT('Ctrl Pts',(21.9865635303682,-3.13696509633072,-3.01828832693899));
#37800=CARTESIAN_POINT('Ctrl Pts',(22.1829088259205,0.789046142938758,-4.28112376882329));
#37801=CARTESIAN_POINT('Ctrl Pts',(22.3792541214728,4.00688260024406,-1.70161873979572));
#37802=CARTESIAN_POINT('Ctrl Pts',(22.5755994170252,3.62851208849374,2.40510176983027));
#37803=CARTESIAN_POINT('Ctrl Pts',(22.7719447125775,-0.00647503630907179,
4.35322553821067));
#37804=CARTESIAN_POINT('Ctrl Pts',(22.9682900081298,-3.63565076862356,2.3942969732266));
#37805=CARTESIAN_POINT('Ctrl Pts',(23.1646353036822,-4.00180286733272,-1.71353095038872));
#37806=CARTESIAN_POINT('Ctrl Pts',(23.3609805992345,-0.776307098369514,
-4.2834520888624));
#37807=CARTESIAN_POINT('Ctrl Pts',(23.5573258947868,3.14593007128556,-3.00894308592204));
#37808=CARTESIAN_POINT('Ctrl Pts',(23.7536711903391,4.24467157966798,0.966114738857153));
#37809=CARTESIAN_POINT('Ctrl Pts',(23.9500164858915,1.53378874262074,4.0740773925992));
#37810=CARTESIAN_POINT('Ctrl Pts',(24.1463617814438,-2.55368091032178,3.52552525391535));
#37811=CARTESIAN_POINT('Ctrl Pts',(24.3427070769961,-4.3492029335743,-0.18721204861699));
#37812=CARTESIAN_POINT('Ctrl Pts',(24.5390523725485,-2.24128294274079,-3.73192514361042));
#37813=CARTESIAN_POINT('Ctrl Pts',(24.7353976681008,1.87820517559581,-3.92720763720996));
#37814=CARTESIAN_POINT('Ctrl Pts',(24.9317429636531,4.31199016615752,-0.597792037071187));
#37815=CARTESIAN_POINT('Ctrl Pts',(25.1280882592054,2.87573187668868,3.26814636651764));
#37816=CARTESIAN_POINT('Ctrl Pts',(25.3244335547578,-1.14151717871423,4.20089907501512));
#37817=CARTESIAN_POINT('Ctrl Pts',(25.5207788503101,-4.13424607503771,1.36331358487529));
#37818=CARTESIAN_POINT('Ctrl Pts',(25.7171241458625,-3.41645832348522,-2.69785599393702));
#37819=CARTESIAN_POINT('Ctrl Pts',(25.9134694414147,0.36762618057702,-4.33767973969799));
#37820=CARTESIAN_POINT('Ctrl Pts',(26.1098147369671,3.82176350742396,-2.08440360887143));
#37821=CARTESIAN_POINT('Ctrl Pts',(26.3061600325194,3.84583952148144,2.03964025048695));
#37822=CARTESIAN_POINT('Ctrl Pts',(26.5025053280717,0.418246147672995,4.3330918565512));
#37823=CARTESIAN_POINT('Ctrl Pts',(26.6988506236241,-3.38472667816454,2.73756114904763));
#37824=CARTESIAN_POINT('Ctrl Pts',(26.8951959191764,-4.1498812911313,-1.3149508547382));
#37825=CARTESIAN_POINT('Ctrl Pts',(27.0915412147287,-1.19048814359663,-4.18728509855987));
#37826=CARTESIAN_POINT('Ctrl Pts',(27.287886510281,2.83738008319601,-3.30149896851051));
#37827=CARTESIAN_POINT('Ctrl Pts',(27.4842318058334,4.31867250924111,0.547405464360225));
#37828=CARTESIAN_POINT('Ctrl Pts',(27.6805771013857,1.92393598980375,3.90501253734012));
#37829=CARTESIAN_POINT('Ctrl Pts',(27.876922396938,-2.19757035780072,3.75783570775159));
#37830=CARTESIAN_POINT('Ctrl Pts',(28.0732676924903,-4.34669624373498,0.237985187117125));
#37831=CARTESIAN_POINT('Ctrl Pts',(28.2696129880427,-2.59471695542828,-3.49548186039235));
#37832=CARTESIAN_POINT('Ctrl Pts',(28.465958283595,1.48620969244535,-4.09168302153342));
#37833=CARTESIAN_POINT('Ctrl Pts',(28.6623035791473,4.23292180679059,-1.01565563961584));
#37834=CARTESIAN_POINT('Ctrl Pts',(28.8586488746997,3.18119835971342,2.97210052421617));
#37835=CARTESIAN_POINT('Ctrl Pts',(29.054994170252,-0.726927517204469,4.29204271131644));
#37836=CARTESIAN_POINT('Ctrl Pts',(29.2513394658043,-3.9801860331636,1.76049028754586));
#37837=CARTESIAN_POINT('Ctrl Pts',(29.4476847613566,-3.66599725731076,-2.35237064874011));
#37838=CARTESIAN_POINT('Ctrl Pts',(29.644030056909,-0.0518048499186609,
-4.35153881345912));
#37839=CARTESIAN_POINT('Ctrl Pts',(29.7749269206105,2.3732446773952,-3.08360315283289));
#37840=CARTESIAN_POINT('Ctrl Pts',(29.8403753524613,3.05685166691388,-2.07796100757108));
#37841=CARTESIAN_POINT('Ctrl Pts',(18.,-1.74869447533108,3.5228619944509));
#37842=CARTESIAN_POINT('Ctrl Pts',(18.0654484318508,-2.9076445584856,2.94757701002939));
#37843=CARTESIAN_POINT('Ctrl Pts',(18.1963452955523,-4.59482537887781,0.574399724304409));
#37844=CARTESIAN_POINT('Ctrl Pts',(18.3926905911047,-3.00975651390536,-3.52461436233937));
#37845=CARTESIAN_POINT('Ctrl Pts',(18.589035886657,1.28055356420065,-4.45033921309645));
#37846=CARTESIAN_POINT('Ctrl Pts',(18.7853811822093,4.41954015077335,-1.38672939105928));
#37847=CARTESIAN_POINT('Ctrl Pts',(18.9817264777616,3.59299056384847,2.92396401486012));
#37848=CARTESIAN_POINT('Ctrl Pts',(19.178071773314,-0.458825554726167,4.60910475875735));
#37849=CARTESIAN_POINT('Ctrl Pts',(19.3744170688663,-4.09856982612836,2.15819318406819));
#37850=CARTESIAN_POINT('Ctrl Pts',(19.5707623644186,-4.05995707399241,-2.23004836909123));
#37851=CARTESIAN_POINT('Ctrl Pts',(19.7671076599709,-0.37743078428812,-4.61663263431879));
#37852=CARTESIAN_POINT('Ctrl Pts',(19.9634529555233,3.64380556037334,-2.85984319112657));
#37853=CARTESIAN_POINT('Ctrl Pts',(20.1597982510756,4.39471822347621,1.46372222413157));
#37854=CARTESIAN_POINT('Ctrl Pts',(20.3561435466279,1.20132883759377,4.47356272690641));
#37855=CARTESIAN_POINT('Ctrl Pts',(20.5524888421803,-3.07025713168235,3.4683593482684));
#37856=CARTESIAN_POINT('Ctrl Pts',(20.7488341377326,-4.58626702982487,-0.649728515655752));
#37857=CARTESIAN_POINT('Ctrl Pts',(20.9451794332849,-1.98606680659531,-4.18467704303101));
#37858=CARTESIAN_POINT('Ctrl Pts',(21.1415247288372,2.39664248654891,-3.96384838890765));
#37859=CARTESIAN_POINT('Ctrl Pts',(21.3378700243896,4.62834765137447,-0.185435461772265));
#37860=CARTESIAN_POINT('Ctrl Pts',(21.5342153199419,2.70607616170119,3.75940674568056));
#37861=CARTESIAN_POINT('Ctrl Pts',(21.7305606154942,-1.64491873905791,4.33015362850052));
#37862=CARTESIAN_POINT('Ctrl Pts',(21.9269059110466,-4.51958687163654,1.01455527800489));
#37863=CARTESIAN_POINT('Ctrl Pts',(22.1232512065988,-3.33789211332263,-3.21161393029448));
#37864=CARTESIAN_POINT('Ctrl Pts',(22.3195965021512,0.83958565578034,-4.5553357545572));
#37865=CARTESIAN_POINT('Ctrl Pts',(22.5159417977035,4.26352905424683,-1.81060980821551));
#37866=CARTESIAN_POINT('Ctrl Pts',(22.7122870932558,3.86092338019503,2.55915191362662));
#37867=CARTESIAN_POINT('Ctrl Pts',(22.9086323888082,-0.00688977147203868,
4.63205574346503));
#37868=CARTESIAN_POINT('Ctrl Pts',(23.1049776843605,-3.86851930280594,2.54765505463652));
#37869=CARTESIAN_POINT('Ctrl Pts',(23.3013229799128,-4.25812395731338,-1.82328501261516));
#37870=CARTESIAN_POINT('Ctrl Pts',(23.4976682754651,-0.826030657527862,
-4.55781320676248));
#37871=CARTESIAN_POINT('Ctrl Pts',(23.6940135710175,3.3474313075052,-3.20167011347485));
#37872=CARTESIAN_POINT('Ctrl Pts',(23.8903588665698,4.51654875152767,1.02799574377413));
#37873=CARTESIAN_POINT('Ctrl Pts',(24.0867041621221,1.63203006418057,4.33502776735682));
#37874=CARTESIAN_POINT('Ctrl Pts',(24.2830494576745,-2.71724775658992,3.75134009432509));
#37875=CARTESIAN_POINT('Ctrl Pts',(24.4793947532267,-4.62777548535616,-0.199203243073542));
#37876=CARTESIAN_POINT('Ctrl Pts',(24.6757400487791,-2.38484026075065,-3.97096018662691));
#37877=CARTESIAN_POINT('Ctrl Pts',(24.8720853443314,1.99850685305871,-4.17875079801063));
#37878=CARTESIAN_POINT('Ctrl Pts',(25.0684306398838,4.58817918796009,-0.636081456016511));
#37879=CARTESIAN_POINT('Ctrl Pts',(25.2647759354361,3.05992653933489,3.47747572797129));
#37880=CARTESIAN_POINT('Ctrl Pts',(25.4611212309884,-1.2146329560725,4.4699725565193));
#37881=CARTESIAN_POINT('Ctrl Pts',(25.6574665265407,-4.39905033834923,1.45063573332825));
#37882=CARTESIAN_POINT('Ctrl Pts',(25.8538118220931,-3.63528727393098,-2.87065745665316));
#37883=CARTESIAN_POINT('Ctrl Pts',(26.0501571176454,0.391173153387717,-4.61551421473986));
#37884=CARTESIAN_POINT('Ctrl Pts',(26.2465024131977,4.06655282372633,-2.21791258537474));
#37885=CARTESIAN_POINT('Ctrl Pts',(26.44284770875,4.09217094027366,2.1702820710626));
#37886=CARTESIAN_POINT('Ctrl Pts',(26.6391930043024,0.445035400418794,4.61063247123866));
#37887=CARTESIAN_POINT('Ctrl Pts',(26.8355382998547,-3.60152317219375,2.9129057826728));
#37888=CARTESIAN_POINT('Ctrl Pts',(27.031883595407,-4.41568701197684,-1.39917530245121));
#37889=CARTESIAN_POINT('Ctrl Pts',(27.2282288909594,-1.26674057998394,-4.45548658576556));
#37890=CARTESIAN_POINT('Ctrl Pts',(27.4245741865117,3.0191182596442,-3.51296461093051));
#37891=CARTESIAN_POINT('Ctrl Pts',(27.620919482064,4.59528954449653,0.582467552608381));
#37892=CARTESIAN_POINT('Ctrl Pts',(27.8172647776163,2.04716679009758,4.15513407084441));
#37893=CARTESIAN_POINT('Ctrl Pts',(28.0136100731686,-2.33832782339674,3.99853035876552));
#37894=CARTESIAN_POINT('Ctrl Pts',(28.209955368721,-4.62510823851462,0.253228472352165));
#37895=CARTESIAN_POINT('Ctrl Pts',(28.4063006642733,-2.76091221797754,-3.71937237928253));
#37896=CARTESIAN_POINT('Ctrl Pts',(28.6026459598257,1.58140350906662,-4.35376106153289));
#37897=CARTESIAN_POINT('Ctrl Pts',(28.798991255378,4.50404638920727,-1.08070980875459));
#37898=CARTESIAN_POINT('Ctrl Pts',(28.9953365509303,3.38495857930413,3.16246773398503));
#37899=CARTESIAN_POINT('Ctrl Pts',(29.1916818464826,-0.773488244887422,
4.56695407064121));
#37900=CARTESIAN_POINT('Ctrl Pts',(29.3880271420349,-4.23512253457759,1.8732521612223));
#37901=CARTESIAN_POINT('Ctrl Pts',(29.5843724375873,-3.90080952668333,-2.50304329022518));
#37902=CARTESIAN_POINT('Ctrl Pts',(29.7807177331396,-0.0551230232614539,
-4.6302609816259));
#37903=CARTESIAN_POINT('Ctrl Pts',(29.9116145968412,2.52525432971127,-3.28111226245297));
#37904=CARTESIAN_POINT('Ctrl Pts',(29.9770630286919,3.25264730631648,-2.21105732641923));
#37905=CARTESIAN_POINT('Ctrl Pts',(29.470836477965,-3.9278981228736,0.00143380487199485));
#37906=CARTESIAN_POINT('Ctrl Pts',(29.50289098531,-3.92594160481835,-0.634441539882881));
#37907=CARTESIAN_POINT('Ctrl Pts',(29.534945492655,-3.77702635946811,-1.27129224464512));
#37908=CARTESIAN_POINT('Ctrl Pts',(29.567,-3.48672441430162,-1.83213518456555));
#37909=CARTESIAN_POINT('',(18.,-1.871586531739,-2.6236008493506));
#37910=CARTESIAN_POINT('Ctrl Pts',(18.,-1.87548423476387,-2.62663505508783));
#37911=CARTESIAN_POINT('Ctrl Pts',(18.,-1.95820209882815,-2.5806971131868));
#37912=CARTESIAN_POINT('Ctrl Pts',(18.,-2.03859008372278,-2.53101906286817));
#37913=CARTESIAN_POINT('Ctrl Pts',(18.,-2.11635819108058,-2.47766066360094));
#37914=CARTESIAN_POINT('Ctrl Pts',(18.,-2.20135601840208,-2.41934179535073));
#37915=CARTESIAN_POINT('Ctrl Pts',(18.,-2.28322550321657,-2.35662754124991));
#37916=CARTESIAN_POINT('Ctrl Pts',(18.,-2.3618759087473,-2.28990546259509));
#37917=CARTESIAN_POINT('Ctrl Pts',(18.,-2.4106981454921,-2.24848773438112));
#37918=CARTESIAN_POINT('Ctrl Pts',(18.,-2.45827961310671,-2.20552464637135));
#37919=CARTESIAN_POINT('Ctrl Pts',(18.,-2.50459424286804,-2.16110001301956));
#37920=CARTESIAN_POINT('Ctrl Pts',(18.,-2.51914286810609,-2.14714508462428));
#37921=CARTESIAN_POINT('Ctrl Pts',(18.,-2.53356646013624,-2.13304589193832));
#37922=CARTESIAN_POINT('Ctrl Pts',(18.,-2.54786413133718,-2.11880491015565));
#37923=CARTESIAN_POINT('Ctrl Pts',(18.,-2.5610050207126,-2.10571612362718));
#37924=CARTESIAN_POINT('Ctrl Pts',(18.,-2.57403244485455,-2.09251462753296));
#37925=CARTESIAN_POINT('Ctrl Pts',(18.,-2.58694576270026,-2.07920297048157));
#37926=CARTESIAN_POINT('Ctrl Pts',(18.,-2.66074697646445,-2.00312519873119));
#37927=CARTESIAN_POINT('Ctrl Pts',(18.,-2.73082522813611,-1.92345089854155));
#37928=CARTESIAN_POINT('Ctrl Pts',(18.,-2.79708762582428,-1.8405877306472));
#37929=CARTESIAN_POINT('Ctrl Pts',(18.,-2.86107601659434,-1.76056827839887));
#37930=CARTESIAN_POINT('Ctrl Pts',(18.,-2.92150620456706,-1.67757429735906));
#37931=CARTESIAN_POINT('Ctrl Pts',(18.,-2.97827186634913,-1.5919350994066));
#37932=CARTESIAN_POINT('Ctrl Pts',(18.,-3.0040065994896,-1.55311053828141));
#37933=CARTESIAN_POINT('Ctrl Pts',(18.,-3.0289878389067,-1.51374185880171));
#37934=CARTESIAN_POINT('Ctrl Pts',(18.,-3.05320386225338,-1.47385768533847));
#37935=CARTESIAN_POINT('Ctrl Pts',(18.,-3.06286630348485,-1.45794349180484));
#37936=CARTESIAN_POINT('Ctrl Pts',(18.,-3.07240777935416,-1.44194571330402));
#37937=CARTESIAN_POINT('Ctrl Pts',(18.,-3.08182473371469,-1.42587083068939));
#37938=CARTESIAN_POINT('Ctrl Pts',(18.,-3.13788269968003,-1.33017904032833));
#37939=CARTESIAN_POINT('Ctrl Pts',(18.,-3.1893801972824,-1.23201678777164));
#37940=CARTESIAN_POINT('Ctrl Pts',(18.,-3.23622158101597,-1.13181604397664));
#37941=CARTESIAN_POINT('Ctrl Pts',(18.,-3.2838680580919,-1.02989308479643));
#37942=CARTESIAN_POINT('Ctrl Pts',(18.,-3.32669756400407,-0.925860308419108));
#37943=CARTESIAN_POINT('Ctrl Pts',(18.,-3.36457639323085,-0.820129668363867));
#37944=CARTESIAN_POINT('Ctrl Pts',(18.,-3.40248383253285,-0.714319169410486));
#37945=CARTESIAN_POINT('Ctrl Pts',(18.,-3.43543362560168,-0.60680744101958));
#37946=CARTESIAN_POINT('Ctrl Pts',(18.,-3.46325088941741,-0.497976121629401));
#37947=CARTESIAN_POINT('Ctrl Pts',(18.,-3.48290184612153,-0.421094385181289));
#37948=CARTESIAN_POINT('Ctrl Pts',(18.,-3.49999061070311,-0.343553440328808));
#37949=CARTESIAN_POINT('Ctrl Pts',(18.,-3.51444110805291,-0.265481772395751));
#37950=CARTESIAN_POINT('Ctrl Pts',(18.,-3.51875517528347,-0.242174171549102));
#37951=CARTESIAN_POINT('Ctrl Pts',(18.,-3.5228340150811,-0.218819245089493));
#37952=CARTESIAN_POINT('Ctrl Pts',(18.,-3.52667537469033,-0.195420359771128));
#37953=CARTESIAN_POINT('Ctrl Pts',(18.,-3.52997474417659,-0.175322900515618));
#37954=CARTESIAN_POINT('Ctrl Pts',(18.,-3.53309932126695,-0.155189617330016));
#37955=CARTESIAN_POINT('Ctrl Pts',(18.,-3.53604413380429,-0.135048340030048));
#37956=CARTESIAN_POINT('Ctrl Pts',(18.,-3.55280836711581,-0.0203880458457306));
#37957=CARTESIAN_POINT('Ctrl Pts',(18.,-3.56377865807533,0.0946897512260063));
#37958=CARTESIAN_POINT('Ctrl Pts',(18.,-3.56881809050027,0.209758022820131));
#37959=CARTESIAN_POINT('Ctrl Pts',(18.,-3.57221961033072,0.287426890001854));
#37960=CARTESIAN_POINT('Ctrl Pts',(18.,-3.57291822578798,0.365092165535591));
#37961=CARTESIAN_POINT('Ctrl Pts',(18.,-3.57086003709278,0.442628950421449));
#37962=CARTESIAN_POINT('Ctrl Pts',(18.,-3.56790903708174,0.55380002700326));
#37963=CARTESIAN_POINT('Ctrl Pts',(18.,-3.55929342003541,0.664706972490521));
#37964=CARTESIAN_POINT('Ctrl Pts',(18.,-3.54527493044651,0.775065658256069));
#37965=CARTESIAN_POINT('Ctrl Pts',(18.,-3.53100071169589,0.887437537669873));
#37966=CARTESIAN_POINT('Ctrl Pts',(18.,-3.5111245897341,0.99924165895933));
#37967=CARTESIAN_POINT('Ctrl Pts',(18.,-3.48586888045152,1.1101799969906));
#37968=CARTESIAN_POINT('Ctrl Pts',(18.,-3.47993938872303,1.13622590805053));
#37969=CARTESIAN_POINT('Ctrl Pts',(18.,-3.47371314341635,1.16222407852405));
#37970=CARTESIAN_POINT('Ctrl Pts',(18.,-3.4671926118425,1.18817060124356));
#37971=CARTESIAN_POINT('Ctrl Pts',(18.,-3.46255239536067,1.20663496737776));
#37972=CARTESIAN_POINT('Ctrl Pts',(18.,-3.45776266140388,1.22507464083751));
#37973=CARTESIAN_POINT('Ctrl Pts',(18.,-3.45282996231712,1.24346791507144));
#37974=CARTESIAN_POINT('Ctrl Pts',(18.,-3.42331447864212,1.35352660217804));
#37975=CARTESIAN_POINT('Ctrl Pts',(18.,-3.38864432210052,1.46208840194843));
#37976=CARTESIAN_POINT('Ctrl Pts',(18.,-3.34912202183174,1.56886148963333));
#37977=CARTESIAN_POINT('Ctrl Pts',(18.,-3.30832864479712,1.67906850677204));
#37978=CARTESIAN_POINT('Ctrl Pts',(18.,-3.26236597176655,1.78737060465608));
#37979=CARTESIAN_POINT('Ctrl Pts',(18.,-3.21151133264799,1.8934501250158));
#37980=CARTESIAN_POINT('Ctrl Pts',(18.,-3.16017558190922,2.00053321340384));
#37981=CARTESIAN_POINT('Ctrl Pts',(18.,-3.10385460122732,2.10535227079503));
#37982=CARTESIAN_POINT('Ctrl Pts',(18.,-3.04278075082353,2.20757233088601));
#37983=CARTESIAN_POINT('Ctrl Pts',(18.,-3.0029883232406,2.27417340993702));
#37984=CARTESIAN_POINT('Ctrl Pts',(18.,-2.96117717331697,2.33967099054269));
#37985=CARTESIAN_POINT('Ctrl Pts',(18.,-2.91740050634391,2.40396807347353));
#37986=CARTESIAN_POINT('Ctrl Pts',(18.,-2.90268894811113,2.4255757093476));
#37987=CARTESIAN_POINT('Ctrl Pts',(18.,-2.88775534320413,2.4470477289152));
#37988=CARTESIAN_POINT('Ctrl Pts',(18.,-2.87260150486414,2.46838032818946));
#37989=CARTESIAN_POINT('Ctrl Pts',(18.,-2.86324620498797,2.48155011784085));
#37990=CARTESIAN_POINT('Ctrl Pts',(18.,-2.85380696612941,2.49466676929328));
#37991=CARTESIAN_POINT('Ctrl Pts',(18.,-2.84428419596223,2.50772937397784));
#37992=CARTESIAN_POINT('Ctrl Pts',(18.,-2.83435634685015,2.52134763484544));
#37993=CARTESIAN_POINT('Ctrl Pts',(18.,-2.8243432924092,2.53489947693834));
#37994=CARTESIAN_POINT('Ctrl Pts',(18.,-2.81424721466029,2.54838219855492));
#37995=CARTESIAN_POINT('Ctrl Pts',(18.,-2.74081393044342,2.64644805671393));
#37996=CARTESIAN_POINT('Ctrl Pts',(18.,-2.66296950811265,2.74088992939784));
#37997=CARTESIAN_POINT('Ctrl Pts',(18.,-2.58100499690223,2.83137492858441));
#37998=CARTESIAN_POINT('Ctrl Pts',(18.,-2.49888770204909,2.92202859378974));
#37999=CARTESIAN_POINT('Ctrl Pts',(18.,-2.41263455998783,3.0087114479034));
#38000=CARTESIAN_POINT('Ctrl Pts',(18.,-2.32248838717186,3.09107247079346));
#38001=CARTESIAN_POINT('Ctrl Pts',(18.,-2.23401847417333,3.17190199801509));
#38002=CARTESIAN_POINT('Ctrl Pts',(18.,-2.14179846071257,3.24856963213308));
#38003=CARTESIAN_POINT('Ctrl Pts',(18.,-2.04601671705284,3.32071669612736));
#38004=CARTESIAN_POINT('Ctrl Pts',(18.,-1.95040779378605,3.3927335841249));
#38005=CARTESIAN_POINT('Ctrl Pts',(18.,-1.85124960611979,3.4602469787051));
#38006=CARTESIAN_POINT('Ctrl Pts',(18.,-1.74869447533108,3.5228619944509));
#38007=CARTESIAN_POINT('Ctrl Pts',(18.,-1.87548423476386,-2.62663505508783));
#38008=CARTESIAN_POINT('Ctrl Pts',(18.0596576193217,-1.08825137675884,-3.18144260266452));
#38009=CARTESIAN_POINT('Ctrl Pts',(18.1847636704941,1.12516150761905,-3.57262622497546));
#38010=CARTESIAN_POINT('Ctrl Pts',(18.3753181535174,3.62142716015887,-1.1363036219263));
#38011=CARTESIAN_POINT('Ctrl Pts',(18.5716634490697,2.94414196278733,2.39593313727195));
#38012=CARTESIAN_POINT('Ctrl Pts',(18.768008744622,-0.375967469233134,3.77675880022508));
#38013=CARTESIAN_POINT('Ctrl Pts',(18.9310454113565,-2.85246745308514,2.10914645645945));
#38014=CARTESIAN_POINT('Ctrl Pts',(19.0286336462402,-3.21794887923582,0.522734302530077));
#38015=CARTESIAN_POINT('Ctrl Pts',(19.0607734492731,-3.21773234909139,0.000164702477305698));
#38016=CARTESIAN_POINT('Origin',(15.6892265507269,0.,0.));
#38017=CARTESIAN_POINT('',(18.,1.87158653173903,-2.62360084935058));
#38018=CARTESIAN_POINT('Origin',(18.,0.,0.));
#38019=CARTESIAN_POINT('Ctrl Pts',(18.,1.87158653173903,-2.62360084935058));
#38020=CARTESIAN_POINT('Ctrl Pts',(18.0654484318508,2.73469795288145,-2.00788687304197));
#38021=CARTESIAN_POINT('Ctrl Pts',(18.1963452955523,3.79210558070424,0.130964326648123));
#38022=CARTESIAN_POINT('Ctrl Pts',(18.3926905911047,1.97820456802146,3.24194700629428));
#38023=CARTESIAN_POINT('Ctrl Pts',(18.589035886657,-1.6130627898401,3.43470578559991));
#38024=CARTESIAN_POINT('Ctrl Pts',(18.7295478731977,-3.14634040634608,1.36959129364314));
#38025=CARTESIAN_POINT('Ctrl Pts',(18.8046114278877,-3.22658417899954,0.157881475370533));
#38026=CARTESIAN_POINT('Ctrl Pts',(18.8142265507269,-3.22532168306538,0.00249477058570481));
#38027=CARTESIAN_POINT('Ctrl Pts',(17.5899369713081,2.28405859260864,-3.20180657528381));
#38028=CARTESIAN_POINT('Ctrl Pts',(17.6553854031588,3.3373879601839,-2.45039766400564));
#38029=CARTESIAN_POINT('Ctrl Pts',(17.7862822668604,4.6278337596493,0.159827072129988));
#38030=CARTESIAN_POINT('Ctrl Pts',(17.9826275624127,2.41417378513026,3.95642776379034));
#38031=CARTESIAN_POINT('Ctrl Pts',(18.178972857965,-1.96855975562516,4.19166794035048));
#38032=CARTESIAN_POINT('Ctrl Pts',(18.3753181535174,-4.58328013121786,0.669998490589778));
#38033=CARTESIAN_POINT('Ctrl Pts',(18.5716634490697,-3.0850987443137,-3.45562037537898));
#38034=CARTESIAN_POINT('Ctrl Pts',(18.768008744622,1.18230356479204,-4.47845017961223));
#38035=CARTESIAN_POINT('Ctrl Pts',(18.9643540401743,4.38841430798082,-1.48252773677679));
#38036=CARTESIAN_POINT('Ctrl Pts',(19.1606993357267,3.65597544705728,2.84432883466346));
#38037=CARTESIAN_POINT('Ctrl Pts',(19.357044631279,-0.35777220904007,4.61819705076657));
#38038=CARTESIAN_POINT('Ctrl Pts',(19.5533899268313,-4.05039424390049,2.24729253433311));
#38039=CARTESIAN_POINT('Ctrl Pts',(19.7497352223837,-4.10776879369746,-2.14062178900008));
#38040=CARTESIAN_POINT('Ctrl Pts',(19.946080517936,-0.478384358520377,-4.60728745225425));
#38041=CARTESIAN_POINT('Ctrl Pts',(20.1424258134883,3.58035056501647,-2.93889099413954));
#38042=CARTESIAN_POINT('Ctrl Pts',(20.3387711090406,4.42569575871567,1.36718851931307));
#38043=CARTESIAN_POINT('Ctrl Pts',(20.535116404593,1.2989452578469,4.44620281532906));
#38044=CARTESIAN_POINT('Ctrl Pts',(20.7314617001453,-2.99361787167454,3.53471869813215));
#38045=CARTESIAN_POINT('Ctrl Pts',(20.9278069956976,-4.59938688433903,-0.549202649241384));
#38046=CARTESIAN_POINT('Ctrl Pts',(21.1241522912499,-2.07717181620429,-4.14021007709899));
#38047=CARTESIAN_POINT('Ctrl Pts',(21.3204975868023,2.30932036632879,-4.01534836843555));
#38048=CARTESIAN_POINT('Ctrl Pts',(21.5168428823546,4.62318035521908,-0.28668148433296));
#38049=CARTESIAN_POINT('Ctrl Pts',(21.7131881779069,2.78770153983615,3.69928410501389));
#38050=CARTESIAN_POINT('Ctrl Pts',(21.9095334734592,-1.54976015515307,4.36511469950787));
#38051=CARTESIAN_POINT('Ctrl Pts',(22.1058787690116,-4.49630057640805,1.11322233560676));
#38052=CARTESIAN_POINT('Ctrl Pts',(22.3022240645639,-3.40737775223363,-3.13779535441328));
#38053=CARTESIAN_POINT('Ctrl Pts',(22.4985693601163,0.739691972350024,-4.57261835642576));
#38054=CARTESIAN_POINT('Ctrl Pts',(22.6949146556685,4.22288264507703,-1.90348233703615));
#38055=CARTESIAN_POINT('Ctrl Pts',(22.891259951221,3.9160047031351,2.47404325063253));
#38056=CARTESIAN_POINT('Ctrl Pts',(23.0876052467732,0.0944833846028492,
4.63109660154791));
#38057=CARTESIAN_POINT('Ctrl Pts',(23.2839505423256,-3.8118374751247,2.63170627257853));
#38058=CARTESIAN_POINT('Ctrl Pts',(23.4802958378779,-4.29700582080243,-1.72966002961468));
#38059=CARTESIAN_POINT('Ctrl Pts',(23.6766411334302,-0.925579449979732,
-4.53864357752752));
#38060=CARTESIAN_POINT('Ctrl Pts',(23.8729864289826,3.27656136831225,-3.2741607232355));
#38061=CARTESIAN_POINT('Ctrl Pts',(24.0693317245348,4.53796396384225,0.928905757170099));
#38062=CARTESIAN_POINT('Ctrl Pts',(24.2656770200872,1.72651011524057,4.29827240446072));
#38063=CARTESIAN_POINT('Ctrl Pts',(24.4620223156395,-2.63449941555764,3.80990756724199));
#38064=CARTESIAN_POINT('Ctrl Pts',(24.6583676111919,-4.63102610742726,-0.0978776777820504));
#38065=CARTESIAN_POINT('Ctrl Pts',(24.8547129067441,-2.47117238664086,-3.91781697736097));
#38066=CARTESIAN_POINT('Ctrl Pts',(25.0510582022965,1.90657694565293,-4.22148637238187));
#38067=CARTESIAN_POINT('Ctrl Pts',(25.2474034978488,4.57315928208664,-0.736340314681052));
#38068=CARTESIAN_POINT('Ctrl Pts',(25.4437487934011,3.1352970992814,3.40967665095255));
#38069=CARTESIAN_POINT('Ctrl Pts',(25.6400940889535,-1.11651754358445,4.49548344955368));
#38070=CARTESIAN_POINT('Ctrl Pts',(25.8364393845058,-4.36624943602384,1.54656035661739));
#38071=CARTESIAN_POINT('Ctrl Pts',(26.0327846800581,-3.69723983944396,-2.79041212120608));
#38072=CARTESIAN_POINT('Ctrl Pts',(26.2291299756104,0.290069821214124,-4.62296904170733));
#38073=CARTESIAN_POINT('Ctrl Pts',(26.4254752711628,4.01704008353218,-2.30637663962979));
#38074=CARTESIAN_POINT('Ctrl Pts',(26.6218205667151,4.13868613388374,2.08020560116578));
#38075=CARTESIAN_POINT('Ctrl Pts',(26.8181658622674,0.545832179724393,4.59978854162153));
#38076=CARTESIAN_POINT('Ctrl Pts',(27.0145111578198,-3.5369133624434,2.99102562851232));
#38077=CARTESIAN_POINT('Ctrl Pts',(27.2108564533721,-4.44524670958994,-1.30220234720116));
#38078=CARTESIAN_POINT('Ctrl Pts',(27.4072017489244,-1.36394995233954,-4.42669929332562));
#38079=CARTESIAN_POINT('Ctrl Pts',(27.6035470444767,2.94152523715434,-3.57819040089757));
#38080=CARTESIAN_POINT('Ctrl Pts',(27.799892340029,4.60691446598188,0.481751031547769));
#38081=CARTESIAN_POINT('Ctrl Pts',(27.9962376355814,2.13765158660013,4.1093562371118));
#38082=CARTESIAN_POINT('Ctrl Pts',(28.1925829311337,-2.25034069347583,4.04870786697312));
#38083=CARTESIAN_POINT('Ctrl Pts',(28.388928226686,-4.61830214982256,0.354461540273715));
#38084=CARTESIAN_POINT('Ctrl Pts',(28.5852735222383,-2.84195199611733,-3.65820383421496));
#38085=CARTESIAN_POINT('Ctrl Pts',(28.7816188177907,1.48633510618651,-4.387044869924));
#38086=CARTESIAN_POINT('Ctrl Pts',(28.977964113343,4.47816070641504,-1.17956954909381));
#38087=CARTESIAN_POINT('Ctrl Pts',(29.1743094088954,3.45564326691785,3.08870285503582));
#38088=CARTESIAN_POINT('Ctrl Pts',(29.3706547044476,-0.678183987680962,
4.58066113992167));
#38089=CARTESIAN_POINT('Ctrl Pts',(29.5015515681492,-3.01258675481066,2.84023382017821));
#38090=CARTESIAN_POINT('Ctrl Pts',(29.567,-3.56151197810524,1.66856867698424));
#38091=CARTESIAN_POINT('Ctrl Pts',(17.7266246475387,2.1465679056521,-3.00907133330607));
#38092=CARTESIAN_POINT('Ctrl Pts',(17.7920730793895,3.13649129108308,-2.30289406701775));
#38093=CARTESIAN_POINT('Ctrl Pts',(17.9229699430911,4.34925770000094,0.150206156969366));
#38094=CARTESIAN_POINT('Ctrl Pts',(18.1193152386434,2.26885071276066,3.71826751129165));
#38095=CARTESIAN_POINT('Ctrl Pts',(18.3156605341957,-1.85006076703014,3.93934722210029));
#38096=CARTESIAN_POINT('Ctrl Pts',(18.512005829748,-4.30738601195373,0.629667409316655));
#38097=CARTESIAN_POINT('Ctrl Pts',(18.7083511253003,-2.899388821172,-3.24760661390658));
#38098=CARTESIAN_POINT('Ctrl Pts',(18.9046964208527,1.11113388033629,-4.20886638097933));
#38099=CARTESIAN_POINT('Ctrl Pts',(19.101041716405,4.12425028880603,-1.3932858243227));
#38100=CARTESIAN_POINT('Ctrl Pts',(19.2973870119573,3.43590115590782,2.67311224386597));
#38101=CARTESIAN_POINT('Ctrl Pts',(19.4937323075096,-0.336235832103842,
4.34020108031933));
#38102=CARTESIAN_POINT('Ctrl Pts',(19.690077603062,-3.80657760590318,2.11201500890636));
#38103=CARTESIAN_POINT('Ctrl Pts',(19.8864228986143,-3.86049844996293,-2.01176539221754));
#38104=CARTESIAN_POINT('Ctrl Pts',(20.0827681941666,-0.449587639252706,
-4.32994819359135));
#38105=CARTESIAN_POINT('Ctrl Pts',(20.2791134897189,3.36482857257619,-2.76198216045975));
#38106=CARTESIAN_POINT('Ctrl Pts',(20.4754587852713,4.15928755356033,1.28488954093846));
#38107=CARTESIAN_POINT('Ctrl Pts',(20.6718040808236,1.22075423577842,4.17856017191967));
#38108=CARTESIAN_POINT('Ctrl Pts',(20.868149376376,-2.81341471095273,3.32194355148002));
#38109=CARTESIAN_POINT('Ctrl Pts',(21.0644946719282,-4.32252320651873,-0.516142967774858));
#38110=CARTESIAN_POINT('Ctrl Pts',(21.2608399674806,-1.95213483998095,-3.89098690502851));
#38111=CARTESIAN_POINT('Ctrl Pts',(21.4571852630329,2.17030902721659,-3.77364134422321));
#38112=CARTESIAN_POINT('Ctrl Pts',(21.6535305585852,4.34488441087682,-0.269424468971688));
#38113=CARTESIAN_POINT('Ctrl Pts',(21.8498758541376,2.6198936731806,3.47660281544816));
#38114=CARTESIAN_POINT('Ctrl Pts',(22.0462211496899,-1.45647113488039,4.10235321842256));
#38115=CARTESIAN_POINT('Ctrl Pts',(22.2425664452422,-4.22564225922916,1.04621104957702));
#38116=CARTESIAN_POINT('Ctrl Pts',(22.4389117407945,-3.20226799305709,-2.94891331776001));
#38117=CARTESIAN_POINT('Ctrl Pts',(22.6352570363469,0.695165637630007,-4.29736603100399));
#38118=CARTESIAN_POINT('Ctrl Pts',(22.8316023318991,3.96868293335011,-1.78890073436812));
#38119=CARTESIAN_POINT('Ctrl Pts',(23.0279476274516,3.68027774827436,2.32511628913057));
#38120=CARTESIAN_POINT('Ctrl Pts',(23.2242929230038,0.0887958836354571,
4.35232413258873));
#38121=CARTESIAN_POINT('Ctrl Pts',(23.4206382185562,-3.58238094773194,2.47328866260319));
#38122=CARTESIAN_POINT('Ctrl Pts',(23.6169835141085,-4.03834420674827,-1.62554179620221));
#38123=CARTESIAN_POINT('Ctrl Pts',(23.8133288096608,-0.869863473681043,
-4.2654363903982));
#38124=CARTESIAN_POINT('Ctrl Pts',(24.0096741052132,3.07932620331151,-3.07707006693597));
#38125=CARTESIAN_POINT('Ctrl Pts',(24.2060194007655,4.26479768658833,0.872989551217906));
#38126=CARTESIAN_POINT('Ctrl Pts',(24.4023646963178,1.62258149337857,4.03953454741621));
#38127=CARTESIAN_POINT('Ctrl Pts',(24.5987099918701,-2.47591367016399,3.5805672121582));
#38128=CARTESIAN_POINT('Ctrl Pts',(24.7950552874225,-4.3522578819166,-0.091985854691575));
#38129=CARTESIAN_POINT('Ctrl Pts',(24.9914005829748,-2.32241823903413,-3.68198093124091));
#38130=CARTESIAN_POINT('Ctrl Pts',(25.1877458785272,1.7918090606076,-3.96737071037795));
#38131=CARTESIAN_POINT('Ctrl Pts',(25.3840911740794,4.29787439522318,-0.692015735606349));
#38132=CARTESIAN_POINT('Ctrl Pts',(25.5804364696318,2.94656544704267,3.20442850777609));
#38133=CARTESIAN_POINT('Ctrl Pts',(25.7767817651841,-1.04930789994255,4.22487431996257));
#38134=CARTESIAN_POINT('Ctrl Pts',(25.9731270607364,-4.10341964858966,1.45346395071116));
#38135=CARTESIAN_POINT('Ctrl Pts',(26.1694723562888,-3.4746816060373,-2.62244108899263));
#38136=CARTESIAN_POINT('Ctrl Pts',(26.3658176518411,0.272608842273773,-4.34468581754659));
#38137=CARTESIAN_POINT('Ctrl Pts',(26.5621629473934,3.77523122521125,-2.16754250044026));
#38138=CARTESIAN_POINT('Ctrl Pts',(26.7585082429457,3.88955469676272,1.95498600389246));
#38139=CARTESIAN_POINT('Ctrl Pts',(26.9548535384981,0.512975386297035,4.32290068572809));
#38140=CARTESIAN_POINT('Ctrl Pts',(27.1511988340504,-3.32400610626277,2.81097850988778));
#38141=CARTESIAN_POINT('Ctrl Pts',(27.3475441296027,-4.1776616197106,-1.22381526210078));
#38142=CARTESIAN_POINT('Ctrl Pts',(27.543889425155,-1.28184592202771,-4.16023067962239));
#38143=CARTESIAN_POINT('Ctrl Pts',(27.7402347207074,2.76445783316343,-3.36279844121984));
#38144=CARTESIAN_POINT('Ctrl Pts',(27.9365800162597,4.32959765951831,0.452751652773583));
#38145=CARTESIAN_POINT('Ctrl Pts',(28.132925311812,2.00897398346573,3.86199033598386));
#38146=CARTESIAN_POINT('Ctrl Pts',(28.3292706073643,-2.11487968173407,3.80499274174914));
#38147=CARTESIAN_POINT('Ctrl Pts',(28.5256159029167,-4.34029985285574,0.333124451623868));
#38148=CARTESIAN_POINT('Ctrl Pts',(28.721961198469,-2.67087848096839,-3.43799540356397));
#38149=CARTESIAN_POINT('Ctrl Pts',(28.9183064940213,1.39686400616373,-4.12296328514024));
#38150=CARTESIAN_POINT('Ctrl Pts',(29.1146517895736,4.20859433284684,-1.10856444084362));
#38151=CARTESIAN_POINT('Ctrl Pts',(29.310997085126,3.24762812747141,2.90277597964053));
#38152=CARTESIAN_POINT('Ctrl Pts',(29.5073423806783,-0.637360174031477,
4.3049246728796));
#38153=CARTESIAN_POINT('Ctrl Pts',(29.6382392443799,-2.83124174738595,2.6692637319689));
#38154=CARTESIAN_POINT('Ctrl Pts',(29.7036876762306,-3.34712398908505,1.56812788515203));
#38155=CARTESIAN_POINT('Ctrl Pts',(17.8633123237694,2.00907721869556,-2.81633609132832));
#38156=CARTESIAN_POINT('Ctrl Pts',(17.9287607556201,2.93559462198226,-2.15539047002986));
#38157=CARTESIAN_POINT('Ctrl Pts',(18.0596576193217,4.07068164035259,0.140585241808746));
#38158=CARTESIAN_POINT('Ctrl Pts',(18.256002914874,2.12352764039106,3.48010725879296));
#38159=CARTESIAN_POINT('Ctrl Pts',(18.4523482104263,-1.73156177843512,3.6870265038501));
#38160=CARTESIAN_POINT('Ctrl Pts',(18.6486935059787,-4.0314918926896,0.589336328043536));
#38161=CARTESIAN_POINT('Ctrl Pts',(18.845038801531,-2.7136788980303,-3.03959285243419));
#38162=CARTESIAN_POINT('Ctrl Pts',(19.0413840970833,1.03996419588054,-3.93928258234643));
#38163=CARTESIAN_POINT('Ctrl Pts',(19.2377293926356,3.86008626963124,-1.3040439118686));
#38164=CARTESIAN_POINT('Ctrl Pts',(19.434074688188,3.21582686475836,2.50189565306848));
#38165=CARTESIAN_POINT('Ctrl Pts',(19.6304199837403,-0.314699455167615,
4.06220510987209));
#38166=CARTESIAN_POINT('Ctrl Pts',(19.8267652792926,-3.56276096790587,1.97673748347961));
#38167=CARTESIAN_POINT('Ctrl Pts',(20.0231105748449,-3.61322810622841,-1.882908995435));
#38168=CARTESIAN_POINT('Ctrl Pts',(20.2194558703973,-0.420790919985035,
-4.05260893492845));
#38169=CARTESIAN_POINT('Ctrl Pts',(20.4158011659496,3.14930658013591,-2.58507332677998));
#38170=CARTESIAN_POINT('Ctrl Pts',(20.6121464615019,3.89287934840499,1.20259056256386));
#38171=CARTESIAN_POINT('Ctrl Pts',(20.8084917570543,1.14256321370995,3.91091752851028));
#38172=CARTESIAN_POINT('Ctrl Pts',(21.0048370526065,-2.63321155023091,3.10916840482789));
#38173=CARTESIAN_POINT('Ctrl Pts',(21.2011823481589,-4.04565952869842,-0.483083286308333));
#38174=CARTESIAN_POINT('Ctrl Pts',(21.3975276437112,-1.8270978637576,-3.64176373295804));
#38175=CARTESIAN_POINT('Ctrl Pts',(21.5938729392636,2.03129768810438,-3.53193432001087));
#38176=CARTESIAN_POINT('Ctrl Pts',(21.7902182348159,4.06658846653455,-0.252167453610417));
#38177=CARTESIAN_POINT('Ctrl Pts',(21.9865635303682,2.45208580652506,3.25392152588244));
#38178=CARTESIAN_POINT('Ctrl Pts',(22.1829088259205,-1.36318211460772,3.83959173733726));
#38179=CARTESIAN_POINT('Ctrl Pts',(22.3792541214729,-3.95498394205026,0.979199763547288));
#38180=CARTESIAN_POINT('Ctrl Pts',(22.5755994170252,-2.99715823388054,-2.76003128110674));
#38181=CARTESIAN_POINT('Ctrl Pts',(22.7719447125776,0.650639302909993,-4.02211370558222));
#38182=CARTESIAN_POINT('Ctrl Pts',(22.9682900081298,3.71448322162319,-1.67431913170009));
#38183=CARTESIAN_POINT('Ctrl Pts',(23.1646353036822,3.44455079341363,2.17618932762861));
#38184=CARTESIAN_POINT('Ctrl Pts',(23.3609805992344,0.0831083826680549,
4.07355166362955));
#38185=CARTESIAN_POINT('Ctrl Pts',(23.5573258947869,-3.35292442033917,2.31487105262785));
#38186=CARTESIAN_POINT('Ctrl Pts',(23.7536711903391,-3.77968259269412,-1.52142356278974));
#38187=CARTESIAN_POINT('Ctrl Pts',(23.9500164858915,-0.814147497382348,
-3.99222920326887));
#38188=CARTESIAN_POINT('Ctrl Pts',(24.1463617814438,2.88209103831078,-2.87997941063644));
#38189=CARTESIAN_POINT('Ctrl Pts',(24.3427070769961,3.99163140933442,0.817073345265716));
#38190=CARTESIAN_POINT('Ctrl Pts',(24.5390523725485,1.51865287151657,3.7807966903717));
#38191=CARTESIAN_POINT('Ctrl Pts',(24.7353976681007,-2.31732792477034,3.3512268570744));
#38192=CARTESIAN_POINT('Ctrl Pts',(24.9317429636531,-4.07348965640595,-0.0860940316010964));
#38193=CARTESIAN_POINT('Ctrl Pts',(25.1280882592054,-2.17366409142741,-3.44614488512086));
#38194=CARTESIAN_POINT('Ctrl Pts',(25.3244335547578,1.67704117556227,-3.71325504837403));
#38195=CARTESIAN_POINT('Ctrl Pts',(25.5207788503101,4.02258950835972,-0.647691156531652));
#38196=CARTESIAN_POINT('Ctrl Pts',(25.7171241458624,2.75783379480394,2.99918036459964));
#38197=CARTESIAN_POINT('Ctrl Pts',(25.9134694414148,-0.982098256300655,
3.95426519037146));
#38198=CARTESIAN_POINT('Ctrl Pts',(26.1098147369671,-3.84058986115548,1.36036754480492));
#38199=CARTESIAN_POINT('Ctrl Pts',(26.3061600325194,-3.25212337263064,-2.45447005677918));
#38200=CARTESIAN_POINT('Ctrl Pts',(26.5025053280717,0.255147863333422,-4.06640259338584));
#38201=CARTESIAN_POINT('Ctrl Pts',(26.6988506236241,3.53342236689032,-2.02870836125074));
#38202=CARTESIAN_POINT('Ctrl Pts',(26.8951959191764,3.64042325964169,1.82976640661915));
#38203=CARTESIAN_POINT('Ctrl Pts',(27.0915412147287,0.480118592869677,4.04601282983465));
#38204=CARTESIAN_POINT('Ctrl Pts',(27.2878865102811,-3.11109885008213,2.63093139126324));
#38205=CARTESIAN_POINT('Ctrl Pts',(27.4842318058334,-3.91007652983126,-1.14542817700039));
#38206=CARTESIAN_POINT('Ctrl Pts',(27.6805771013857,-1.19974189171588,-3.89376206591915));
#38207=CARTESIAN_POINT('Ctrl Pts',(27.876922396938,2.58739042917252,-3.14740648154211));
#38208=CARTESIAN_POINT('Ctrl Pts',(28.0732676924904,4.05228085305474,0.423752273999395));
#38209=CARTESIAN_POINT('Ctrl Pts',(28.2696129880427,1.88029638033132,3.61462443485592));
#38210=CARTESIAN_POINT('Ctrl Pts',(28.465958283595,-1.97941866999231,3.56127761652517));
#38211=CARTESIAN_POINT('Ctrl Pts',(28.6623035791473,-4.06229755588892,0.311787362974019));
#38212=CARTESIAN_POINT('Ctrl Pts',(28.8586488746997,-2.49980496581944,-3.21778697291297));
#38213=CARTESIAN_POINT('Ctrl Pts',(29.0549941702519,1.30739290614095,-3.85888170035648));
#38214=CARTESIAN_POINT('Ctrl Pts',(29.2513394658043,3.93902795927863,-1.03755933259342));
#38215=CARTESIAN_POINT('Ctrl Pts',(29.4476847613566,3.03961298802498,2.71684910424524));
#38216=CARTESIAN_POINT('Ctrl Pts',(29.644030056909,-0.596536360381995,4.02918820583754));
#38217=CARTESIAN_POINT('Ctrl Pts',(29.7749269206105,-2.64989673996124,2.49829364375959));
#38218=CARTESIAN_POINT('Ctrl Pts',(29.8403753524613,-3.13273600006486,1.46768709331983));
#38219=CARTESIAN_POINT('Ctrl Pts',(18.,1.87158653173903,-2.62360084935058));
#38220=CARTESIAN_POINT('Ctrl Pts',(18.0654484318508,2.73469795288145,-2.00788687304197));
#38221=CARTESIAN_POINT('Ctrl Pts',(18.1963452955523,3.79210558070424,0.130964326648123));
#38222=CARTESIAN_POINT('Ctrl Pts',(18.3926905911047,1.97820456802146,3.24194700629428));
#38223=CARTESIAN_POINT('Ctrl Pts',(18.589035886657,-1.6130627898401,3.43470578559991));
#38224=CARTESIAN_POINT('Ctrl Pts',(18.7853811822093,-3.75559777342547,0.549005246770418));
#38225=CARTESIAN_POINT('Ctrl Pts',(18.9817264777616,-2.5279689748886,-2.83157909096179));
#38226=CARTESIAN_POINT('Ctrl Pts',(19.178071773314,0.968794511424788,-3.66969878371352));
#38227=CARTESIAN_POINT('Ctrl Pts',(19.3744170688663,3.59592225045646,-1.21480199941451));
#38228=CARTESIAN_POINT('Ctrl Pts',(19.5707623644186,2.99575257360889,2.33067906227099));
#38229=CARTESIAN_POINT('Ctrl Pts',(19.7671076599709,-0.293163078231386,
3.78420913942485));
#38230=CARTESIAN_POINT('Ctrl Pts',(19.9634529555233,-3.31894432990856,1.84145995805286));
#38231=CARTESIAN_POINT('Ctrl Pts',(20.1597982510756,-3.36595776249388,-1.75405259865246));
#38232=CARTESIAN_POINT('Ctrl Pts',(20.3561435466279,-0.391994200717362,
-3.77526967626554));
#38233=CARTESIAN_POINT('Ctrl Pts',(20.5524888421802,2.93378458769563,-2.4081644931002));
#38234=CARTESIAN_POINT('Ctrl Pts',(20.7488341377326,3.62647114324965,1.12029158418925));
#38235=CARTESIAN_POINT('Ctrl Pts',(20.9451794332849,1.06437219164148,3.64327488510088));
#38236=CARTESIAN_POINT('Ctrl Pts',(21.1415247288372,-2.45300838950909,2.89639325817577));
#38237=CARTESIAN_POINT('Ctrl Pts',(21.3378700243895,-3.76879585087811,-0.450023604841809));
#38238=CARTESIAN_POINT('Ctrl Pts',(21.5342153199419,-1.70206088753426,-3.39254056088757));
#38239=CARTESIAN_POINT('Ctrl Pts',(21.7305606154942,1.89228634899218,-3.29022729579853));
#38240=CARTESIAN_POINT('Ctrl Pts',(21.9269059110465,3.78829252219229,-0.234910438249147));
#38241=CARTESIAN_POINT('Ctrl Pts',(22.1232512065989,2.28427793986952,3.03124023631671));
#38242=CARTESIAN_POINT('Ctrl Pts',(22.3195965021511,-1.26989309433504,3.57683025625195));
#38243=CARTESIAN_POINT('Ctrl Pts',(22.5159417977035,-3.68432562487137,0.912188477517553));
#38244=CARTESIAN_POINT('Ctrl Pts',(22.7122870932558,-2.792048474704,-2.57114924445347));
#38245=CARTESIAN_POINT('Ctrl Pts',(22.9086323888082,0.606112968189978,-3.74686138016046));
#38246=CARTESIAN_POINT('Ctrl Pts',(23.1049776843605,3.46028350989628,-1.55973752903206));
#38247=CARTESIAN_POINT('Ctrl Pts',(23.3013229799128,3.2088238385529,2.02726236612665));
#38248=CARTESIAN_POINT('Ctrl Pts',(23.4976682754651,0.0774208817006576,
3.79477919467037));
#38249=CARTESIAN_POINT('Ctrl Pts',(23.6940135710175,-3.1234678929464,2.15645344265251));
#38250=CARTESIAN_POINT('Ctrl Pts',(23.8903588665698,-3.52102097863996,-1.41730532937728));
#38251=CARTESIAN_POINT('Ctrl Pts',(24.0867041621221,-0.758431521083658,
-3.71902201613955));
#38252=CARTESIAN_POINT('Ctrl Pts',(24.2830494576745,2.68485587331004,-2.68288875433691));
#38253=CARTESIAN_POINT('Ctrl Pts',(24.4793947532267,3.71846513208049,0.761157139313524));
#38254=CARTESIAN_POINT('Ctrl Pts',(24.6757400487791,1.41472424965457,3.52205883332719));
#38255=CARTESIAN_POINT('Ctrl Pts',(24.8720853443314,-2.15874217937669,3.12188650199061));
#38256=CARTESIAN_POINT('Ctrl Pts',(25.0684306398838,-3.79472143089529,-0.0802022085106187));
#38257=CARTESIAN_POINT('Ctrl Pts',(25.2647759354361,-2.02490994382068,-3.2103088390008));
#38258=CARTESIAN_POINT('Ctrl Pts',(25.4611212309884,1.56227329051694,-3.45913938637011));
#38259=CARTESIAN_POINT('Ctrl Pts',(25.6574665265407,3.74730462149625,-0.603366577456954));
#38260=CARTESIAN_POINT('Ctrl Pts',(25.8538118220931,2.56910214256522,2.79393222142319));
#38261=CARTESIAN_POINT('Ctrl Pts',(26.0501571176454,-0.914888612658763,
3.68365606078035));
#38262=CARTESIAN_POINT('Ctrl Pts',(26.2465024131977,-3.5777600737213,1.26727113889869));
#38263=CARTESIAN_POINT('Ctrl Pts',(26.44284770875,-3.02956513922398,-2.28649902456573));
#38264=CARTESIAN_POINT('Ctrl Pts',(26.6391930043024,0.237686884393074,-3.7881193692251));
#38265=CARTESIAN_POINT('Ctrl Pts',(26.8355382998547,3.29161350856939,-1.88987422206122));
#38266=CARTESIAN_POINT('Ctrl Pts',(27.0318835954071,3.39129182252066,1.70454680934583));
#38267=CARTESIAN_POINT('Ctrl Pts',(27.2282288909593,0.447261799442319,3.76912497394121));
#38268=CARTESIAN_POINT('Ctrl Pts',(27.4245741865117,-2.89819159390149,2.45088427263869));
#38269=CARTESIAN_POINT('Ctrl Pts',(27.620919482064,-3.64249143995193,-1.0670410919));
#38270=CARTESIAN_POINT('Ctrl Pts',(27.8172647776164,-1.11763786140405,-3.62729345221592));
#38271=CARTESIAN_POINT('Ctrl Pts',(28.0136100731686,2.41032302518161,-2.93201452186437));
#38272=CARTESIAN_POINT('Ctrl Pts',(28.2099553687211,3.77496404659118,0.394752895225204));
#38273=CARTESIAN_POINT('Ctrl Pts',(28.4063006642733,1.75161877719691,3.36725853372798));
#38274=CARTESIAN_POINT('Ctrl Pts',(28.6026459598257,-1.84395765825054,3.31756249130118));
#38275=CARTESIAN_POINT('Ctrl Pts',(28.798991255378,-3.78429525892211,0.290450274324173));
#38276=CARTESIAN_POINT('Ctrl Pts',(28.9953365509303,-2.32873145067049,-2.99757854226198));
#38277=CARTESIAN_POINT('Ctrl Pts',(29.1916818464826,1.21792180611816,-3.59480011557272));
#38278=CARTESIAN_POINT('Ctrl Pts',(29.388027142035,3.66946158571043,-0.966554224343232));
#38279=CARTESIAN_POINT('Ctrl Pts',(29.5843724375873,2.83159784857854,2.53092222884994));
#38280=CARTESIAN_POINT('Ctrl Pts',(29.7807177331396,-0.555712546732512,
3.75345173879546));
#38281=CARTESIAN_POINT('Ctrl Pts',(29.9116145968412,-2.46855173253653,2.32732355555027));
#38282=CARTESIAN_POINT('Ctrl Pts',(29.9770630286919,-2.91834801104467,1.36724630148763));
#38283=CARTESIAN_POINT('Ctrl Pts',(18.,1.75280451302835,3.52727163111204));
#38284=CARTESIAN_POINT('Ctrl Pts',(18.,1.85055634181796,3.46829220042325));
#38285=CARTESIAN_POINT('Ctrl Pts',(18.,1.9453897415748,3.40491824723834));
#38286=CARTESIAN_POINT('Ctrl Pts',(18.,2.03695736150634,3.33713960726484));
#38287=CARTESIAN_POINT('Ctrl Pts',(18.,2.13485777676419,3.26467341229354));
#38288=CARTESIAN_POINT('Ctrl Pts',(18.,2.22902577851624,3.18717173263842));
#38289=CARTESIAN_POINT('Ctrl Pts',(18.,2.31927390895822,3.10504417467128));
#38290=CARTESIAN_POINT('Ctrl Pts',(18.,2.37057338638084,3.05836065020293));
#38291=CARTESIAN_POINT('Ctrl Pts',(18.,2.42060555689673,3.01018185463388));
#38292=CARTESIAN_POINT('Ctrl Pts',(18.,2.46932956368599,2.96057932112694));
#38293=CARTESIAN_POINT('Ctrl Pts',(18.,2.48926772386374,2.94028166246842));
#38294=CARTESIAN_POINT('Ctrl Pts',(18.,2.50898677586689,2.91974557487581));
#38295=CARTESIAN_POINT('Ctrl Pts',(18.,2.52848367972817,2.89897587060429));
#38296=CARTESIAN_POINT('Ctrl Pts',(18.,2.54217196878492,2.88439398018136));
#38297=CARTESIAN_POINT('Ctrl Pts',(18.,2.55574734184337,2.86970051594287));
#38298=CARTESIAN_POINT('Ctrl Pts',(18.,2.56920386940907,2.85490297454373));
#38299=CARTESIAN_POINT('Ctrl Pts',(18.,2.65294903624156,2.76281216083778));
#38300=CARTESIAN_POINT('Ctrl Pts',(18.,2.73215730305588,2.66662713037754));
#38301=CARTESIAN_POINT('Ctrl Pts',(18.,2.80663529425947,2.56679160942941));
#38302=CARTESIAN_POINT('Ctrl Pts',(18.,2.87180353656261,2.4794355285998));
#38303=CARTESIAN_POINT('Ctrl Pts',(18.,2.9333495992658,2.38928354160773));
#38304=CARTESIAN_POINT('Ctrl Pts',(18.,2.99111044370871,2.29661846198891));
#38305=CARTESIAN_POINT('Ctrl Pts',(18.,3.01638081315248,2.25607748965567));
#38306=CARTESIAN_POINT('Ctrl Pts',(18.,3.04092624626456,2.21505537388696));
#38307=CARTESIAN_POINT('Ctrl Pts',(18.,3.06473105776385,2.17357540269015));
#38308=CARTESIAN_POINT('Ctrl Pts',(18.,3.07937622571154,2.14805614391925));
#38309=CARTESIAN_POINT('Ctrl Pts',(18.,3.09374104789547,2.12236358627869));
#38310=CARTESIAN_POINT('Ctrl Pts',(18.,3.10782162822979,2.09650313728402));
#38311=CARTESIAN_POINT('Ctrl Pts',(18.,3.11588415285192,2.08169547298267));
#38312=CARTESIAN_POINT('Ctrl Pts',(18.,3.12385167846963,2.06683599660815));
#38313=CARTESIAN_POINT('Ctrl Pts',(18.,3.1317198130323,2.05193313593188));
#38314=CARTESIAN_POINT('Ctrl Pts',(18.,3.18720095944412,1.94684751639281));
#38315=CARTESIAN_POINT('Ctrl Pts',(18.,3.23780322769338,1.83949826444516));
#38316=CARTESIAN_POINT('Ctrl Pts',(18.,3.28335897157006,1.73026580000651));
#38317=CARTESIAN_POINT('Ctrl Pts',(18.,3.32860687522003,1.62177146744223));
#38318=CARTESIAN_POINT('Ctrl Pts',(18.,3.36887645015951,1.51141841716963));
#38319=CARTESIAN_POINT('Ctrl Pts',(18.,3.40395374640598,1.3995675723142));
#38320=CARTESIAN_POINT('Ctrl Pts',(18.,3.43799986603056,1.29100483654054));
#38321=CARTESIAN_POINT('Ctrl Pts',(18.,3.46715450249439,1.18103033348445));
#38322=CARTESIAN_POINT('Ctrl Pts',(18.,3.49117371118248,1.06997467581908));
#38323=CARTESIAN_POINT('Ctrl Pts',(18.,3.50794056569238,0.992451137106512));
#38324=CARTESIAN_POINT('Ctrl Pts',(18.,3.52220399937057,0.914400770171061));
#38325=CARTESIAN_POINT('Ctrl Pts',(18.,3.53386633916247,0.835939010635201));
#38326=CARTESIAN_POINT('Ctrl Pts',(18.,3.53850288921364,0.804745280930666));
#38327=CARTESIAN_POINT('Ctrl Pts',(18.,3.54272817554279,0.773486566216751));
#38328=CARTESIAN_POINT('Ctrl Pts',(18.,3.54653550521384,0.74217030018733));
#38329=CARTESIAN_POINT('Ctrl Pts',(18.,3.548303818075,0.727625471982788));
#38330=CARTESIAN_POINT('Ctrl Pts',(18.,3.54998159728476,0.713070984488063));
#38331=CARTESIAN_POINT('Ctrl Pts',(18.,3.55156744344722,0.698515996963189));
#38332=CARTESIAN_POINT('Ctrl Pts',(18.,3.56369208352232,0.587235351201648));
#38333=CARTESIAN_POINT('Ctrl Pts',(18.,3.57046471402958,0.47578171671144));
#38334=CARTESIAN_POINT('Ctrl Pts',(18.,3.57169639188583,0.364475115519244));
#38335=CARTESIAN_POINT('Ctrl Pts',(18.,3.57257411457641,0.285155406244404));
#38336=CARTESIAN_POINT('Ctrl Pts',(18.,3.57063694555984,0.205910265097998));
#38337=CARTESIAN_POINT('Ctrl Pts',(18.,3.56580039408165,0.126857466521517));
#38338=CARTESIAN_POINT('Ctrl Pts',(18.,3.55887863429577,0.0137222120711326));
#38339=CARTESIAN_POINT('Ctrl Pts',(18.,3.54602018773888,-0.0990203100151426));
#38340=CARTESIAN_POINT('Ctrl Pts',(18.,3.52743695201649,-0.211010483416101));
#38341=CARTESIAN_POINT('Ctrl Pts',(18.,3.508804805596,-0.323295412673502));
#38342=CARTESIAN_POINT('Ctrl Pts',(18.,3.4844171411277,-0.434824818175472));
#38343=CARTESIAN_POINT('Ctrl Pts',(18.,3.45444382525478,-0.545208161076649));
#38344=CARTESIAN_POINT('Ctrl Pts',(18.,3.44863818325821,-0.56658871750177));
#38345=CARTESIAN_POINT('Ctrl Pts',(18.,3.44262286633546,-0.587926171790228));
#38346=CARTESIAN_POINT('Ctrl Pts',(18.,3.43639894723186,-0.609217525642749));
#38347=CARTESIAN_POINT('Ctrl Pts',(18.,3.4319855878944,-0.624315150429954));
#38348=CARTESIAN_POINT('Ctrl Pts',(18.,3.42746744875845,-0.639389001662136));
#38349=CARTESIAN_POINT('Ctrl Pts',(18.,3.42284901423685,-0.654425291755363));
#38350=CARTESIAN_POINT('Ctrl Pts',(18.,3.39017323849704,-0.760808188545976));
#38351=CARTESIAN_POINT('Ctrl Pts',(18.,3.35243274001992,-0.865480322917389));
#38352=CARTESIAN_POINT('Ctrl Pts',(18.,3.30986573133022,-0.968117196308756));
#38353=CARTESIAN_POINT('Ctrl Pts',(18.,3.26724317972447,-1.07088799386855));
#38354=CARTESIAN_POINT('Ctrl Pts',(18.,3.21978092670367,-1.17161896447357));
#38355=CARTESIAN_POINT('Ctrl Pts',(18.,3.16767339295151,-1.26995725336641));
#38356=CARTESIAN_POINT('Ctrl Pts',(18.,3.11619046641229,-1.36711677212509));
#38357=CARTESIAN_POINT('Ctrl Pts',(18.,3.06017233448318,-1.46194124984198));
#38358=CARTESIAN_POINT('Ctrl Pts',(18.,2.99977200511078,-1.55405385994265));
#38359=CARTESIAN_POINT('Ctrl Pts',(18.,2.96384880635417,-1.60883799166874));
#38360=CARTESIAN_POINT('Ctrl Pts',(18.,2.9263748812984,-1.6626621140883));
#38361=CARTESIAN_POINT('Ctrl Pts',(18.,2.88737785842231,-1.71543935342494));
#38362=CARTESIAN_POINT('Ctrl Pts',(18.,2.869045125242,-1.74025024860087));
#38363=CARTESIAN_POINT('Ctrl Pts',(18.,2.85037574463248,-1.7648296948276));
#38364=CARTESIAN_POINT('Ctrl Pts',(18.,2.83137237441651,-1.78916817371834));
#38365=CARTESIAN_POINT('Ctrl Pts',(18.,2.82197518346086,-1.80120358275932));
#38366=CARTESIAN_POINT('Ctrl Pts',(18.,2.81249924524833,-1.813176259781));
#38367=CARTESIAN_POINT('Ctrl Pts',(18.,2.80294996247512,-1.82507914472327));
#38368=CARTESIAN_POINT('Ctrl Pts',(18.,2.73565253998902,-1.90896329558436));
#38369=CARTESIAN_POINT('Ctrl Pts',(18.,2.66464231294219,-1.98947789681978));
#38370=CARTESIAN_POINT('Ctrl Pts',(18.,2.59009745348758,-2.06630396380742));
#38371=CARTESIAN_POINT('Ctrl Pts',(18.,2.51658282385074,-2.14206827408143));
#38372=CARTESIAN_POINT('Ctrl Pts',(18.,2.43962999231716,-2.21424581024087));
#38373=CARTESIAN_POINT('Ctrl Pts',(18.,2.35938133050909,-2.28248986040027));
#38374=CARTESIAN_POINT('Ctrl Pts',(18.,2.28159477252663,-2.34864011942115));
#38375=CARTESIAN_POINT('Ctrl Pts',(18.,2.20071097356059,-2.41109484295671));
#38376=CARTESIAN_POINT('Ctrl Pts',(18.,2.11684099713627,-2.46949410191337));
#38377=CARTESIAN_POINT('Ctrl Pts',(18.,2.03771972777132,-2.5245868024913));
#38378=CARTESIAN_POINT('Ctrl Pts',(18.,1.95594042011274,-2.57607026124645));
#38379=CARTESIAN_POINT('Ctrl Pts',(18.,1.87158653173906,-2.62360084935056));
#38380=CARTESIAN_POINT('Origin',(23.75,0.,0.));
#38381=CARTESIAN_POINT('Origin',(29.567,0.,0.));
#38382=CARTESIAN_POINT('Origin',(17.,0.,0.));
#38383=CARTESIAN_POINT('',(18.,-8.,-9.79717439317883E-16));
#38384=CARTESIAN_POINT('Origin',(18.,0.,0.));
#38385=CARTESIAN_POINT('',(17.,-9.,-1.10218211923262E-15));
#38386=CARTESIAN_POINT('Origin',(18.,4.,0.));
#38387=CARTESIAN_POINT('Origin',(29.75,0.,0.));
#38388=CARTESIAN_POINT('',(30.,-3.5,-4.28626379701574E-16));
#38389=CARTESIAN_POINT('Origin',(30.,0.,0.));
#38390=CARTESIAN_POINT('',(29.75,-3.75,-4.59242549680257E-16));
#38391=CARTESIAN_POINT('Origin',(30.,0.,0.));
#56613=UNCERTAINTY_MEASURE_WITH_UNIT(LENGTH_MEASURE(0.01),#56640,
'DISTANCE_ACCURACY_VALUE',
'Maximum model space distance between geometric entities at asserted c
onnectivities');
#56617=UNCERTAINTY_MEASURE_WITH_UNIT(LENGTH_MEASURE(0.01),#56640,
'DISTANCE_ACCURACY_VALUE',
'Maximum model space distance between geometric entities at asserted c
onnectivities');
#56635=(
GEOMETRIC_REPRESENTATION_CONTEXT(3)
GLOBAL_UNCERTAINTY_ASSIGNED_CONTEXT((#56613))
GLOBAL_UNIT_ASSIGNED_CONTEXT((#56640,#56642,#56643))
REPRESENTATION_CONTEXT('','3D')
);
#56639=(
GEOMETRIC_REPRESENTATION_CONTEXT(3)
GLOBAL_UNCERTAINTY_ASSIGNED_CONTEXT((#56617))
GLOBAL_UNIT_ASSIGNED_CONTEXT((#56640,#56642,#56643))
REPRESENTATION_CONTEXT('','3D')
);
#56640=(
LENGTH_UNIT()
NAMED_UNIT(*)
SI_UNIT(.MILLI.,.METRE.)
);
#56642=(
NAMED_UNIT(*)
PLANE_ANGLE_UNIT()
SI_UNIT($,.RADIAN.)
);
#56643=(
NAMED_UNIT(*)
SI_UNIT($,.STERADIAN.)
SOLID_ANGLE_UNIT()
);
#56661=SHAPE_DEFINITION_REPRESENTATION(#56682,#56761);
#56682=PRODUCT_DEFINITION_SHAPE('',$,#56783);
#56761=SHAPE_REPRESENTATION('',(#18327),#56635);
#56765=PRODUCT_DEFINITION_CONTEXT('part definition',#56830,'design');
#56783=PRODUCT_DEFINITION('2026-10-26-00-02-52-418',
'15_Cushion_Foot_M8',#56804,#56765);
#56804=PRODUCT_DEFINITION_FORMATION('',$,#56849);
#56830=APPLICATION_CONTEXT(
'Core Data for Automotive Mechanical Design Process');
#56831=PRODUCT_CONTEXT('part definition',#56830,'mechanical');
#56849=PRODUCT('2026-10-26-00-02-52-418','15_Cushion_Foot_M8',$,(#56831));
#56923=COLOUR_RGB('Off White',0.89,0.88,0.83);
#56924=FILL_AREA_STYLE_COLOUR('',#56923);
#56925=FILL_AREA_STYLE('',(#56924));
#56926=SURFACE_STYLE_FILL_AREA(#56925);
#56927=SURFACE_SIDE_STYLE('',(#56926));
#56928=SURFACE_STYLE_USAGE(.BOTH.,#56927);
#56929=PRESENTATION_STYLE_ASSIGNMENT((#56928));
ENDSEC;
END-ISO-10303-21;
